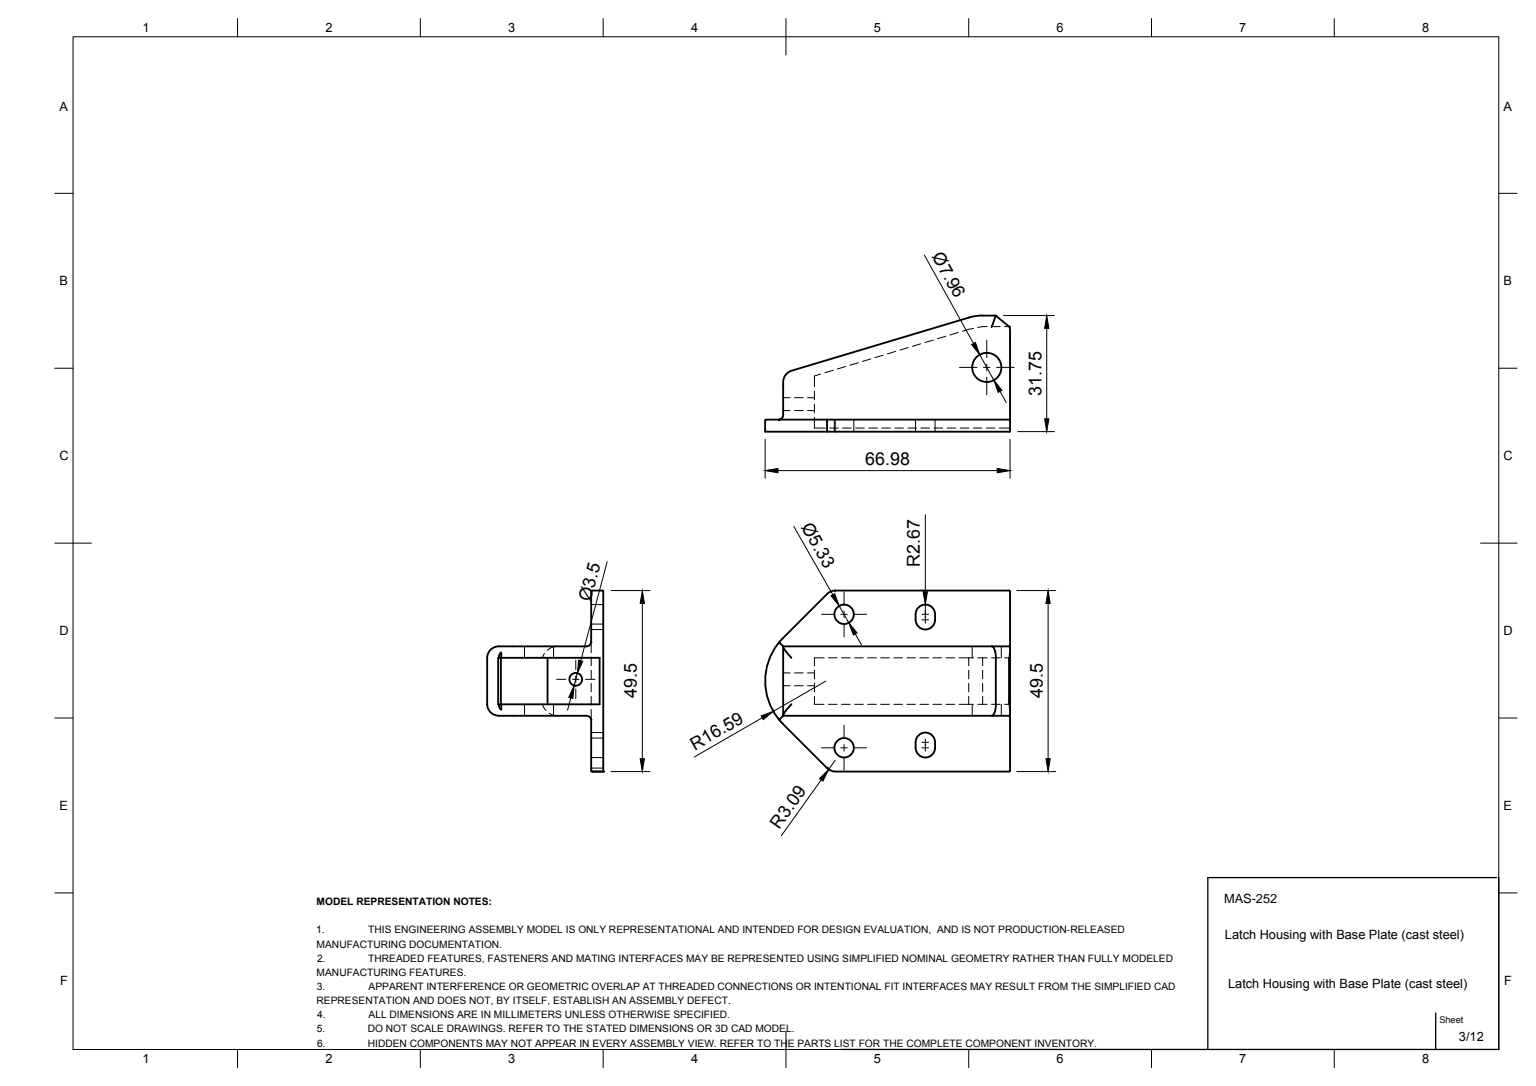
ISO-10303-21;
HEADER;
FILE_DESCRIPTION((''),'2;1');
FILE_NAME('Latch Housing with Base Plate (cast steel).step','2026-10-06T07:01:46+05:00',(''),(''),'','','');
FILE_SCHEMA (('AUTOMOTIVE_DESIGN { 1 0 10303 214 3 1 1 }'));
ENDSEC;
DATA;
#10=MECHANICAL_DESIGN_GEOMETRIC_PRESENTATION_REPRESENTATION('',(#138),#11396);
#108=SHAPE_REPRESENTATION_RELATIONSHIP('SRR','None',#11455,#123) ;
#123=ADVANCED_BREP_SHAPE_REPRESENTATION('',(#153),#11381) ;
#138=STYLED_ITEM('',(#11539),#153) ;
#153=MANIFOLD_SOLID_BREP('Latch Housing with Base Plate (cast steel)',#5569) ;
#168=SPHERICAL_SURFACE('',#5868,0.25) ;
#169=SPHERICAL_SURFACE('',#5870,0.25) ;
#170=B_SPLINE_SURFACE_WITH_KNOTS('',3,3,((#8352,#8353,#8354,#8355,#8356),
(#8357,#8358,#8359,#8360,#8361),(#8362,#8363,#8364,#8365,#8366),(#8367,
#8368,#8369,#8370,#8371),(#8372,#8373,#8374,#8375,#8376)),.UNSPECIFIED.,
 .F.,.F.,.F.,(4,1,4),(4,1,4),(0.,0.5,1.),(0.152021076009298,0.962749790743926,
1.5707963267949),.UNSPECIFIED.) ;
#171=B_SPLINE_SURFACE_WITH_KNOTS('',3,3,((#8498,#8499,#8500,#8501),(#8502,
#8503,#8504,#8505),(#8506,#8507,#8508,#8509),(#8510,#8511,#8512,#8513),
(#8514,#8515,#8516,#8517)),.UNSPECIFIED.,.F.,.F.,.F.,(4,1,4),(4,4),(0.,
0.5,1.),(0.247286151692027,0.297678176745857),.UNSPECIFIED.) ;
#172=B_SPLINE_SURFACE_WITH_KNOTS('',3,3,((#8566,#8567,#8568,#8569),(#8570,
#8571,#8572,#8573),(#8574,#8575,#8576,#8577),(#8578,#8579,#8580,#8581),
(#8582,#8583,#8584,#8585)),.UNSPECIFIED.,.F.,.F.,.F.,(4,1,4),(4,4),(0.,
0.5,1.),(0.268639752323811,0.328790837661693),.UNSPECIFIED.) ;
#173=B_SPLINE_SURFACE_WITH_KNOTS('',3,3,((#8636,#8637,#8638,#8639),(#8640,
#8641,#8642,#8643),(#8644,#8645,#8646,#8647),(#8648,#8649,#8650,#8651),
(#8652,#8653,#8654,#8655)),.UNSPECIFIED.,.F.,.F.,.F.,(4,1,4),(4,4),(0.,
0.5,1.),(8.83098018298437E-16,0.0601510853378708),.UNSPECIFIED.) ;
#174=B_SPLINE_SURFACE_WITH_KNOTS('',3,3,((#8668,#8669,#8670,#8671),(#8672,
#8673,#8674,#8675),(#8676,#8677,#8678,#8679),(#8680,#8681,#8682,#8683),
(#8684,#8685,#8686,#8687)),.UNSPECIFIED.,.F.,.F.,.F.,(4,1,4),(4,4),(0.,
0.5,1.),(1.40103212881273E-16,0.0503920250538296),.UNSPECIFIED.) ;
#175=B_SPLINE_SURFACE_WITH_KNOTS('',3,3,((#8744,#8745,#8746,#8747,#8748),
(#8749,#8750,#8751,#8752,#8753),(#8754,#8755,#8756,#8757,#8758),(#8759,
#8760,#8761,#8762,#8763),(#8764,#8765,#8766,#8767,#8768)),.UNSPECIFIED.,
 .F.,.F.,.F.,(4,1,4),(4,1,4),(0.,0.5,1.),(-1.5707963267949,-0.962749790743935,
-0.152021076009317),.UNSPECIFIED.) ;
#176=TOROIDAL_SURFACE('',#5776,2.915,0.25) ;
#177=TOROIDAL_SURFACE('',#5783,2.915,0.25) ;
#178=TOROIDAL_SURFACE('',#5795,2.915,0.25) ;
#179=TOROIDAL_SURFACE('',#5801,2.915,0.25) ;
#180=TOROIDAL_SURFACE('',#5813,2.915,0.25) ;
#181=TOROIDAL_SURFACE('',#5819,2.915,0.25) ;
#182=TOROIDAL_SURFACE('',#5833,1.52,0.25) ;
#183=TOROIDAL_SURFACE('',#5836,3.05499364382027,0.25) ;
#184=TOROIDAL_SURFACE('',#5838,2.83595375255767,0.25) ;
#185=TOROIDAL_SURFACE('',#5843,16.3358074534161,0.25) ;
#186=TOROIDAL_SURFACE('',#5847,16.3358074534161,0.25) ;
#187=TOROIDAL_SURFACE('',#5850,16.3358074534161,0.25) ;
#188=TOROIDAL_SURFACE('',#5860,1.52,0.25) ;
#189=TOROIDAL_SURFACE('',#5885,10.1848235398934,3.175) ;
#190=TOROIDAL_SURFACE('',#5899,10.1848235398934,3.175) ;
#238=B_SPLINE_CURVE_WITH_KNOTS('',3,(#8214,#8215,#8216,#8217,#8218,#8219,
#8220,#8221,#8222,#8223,#8224,#8225,#8226,#8227,#8228,#8229,#8230,#8231,
#8232,#8233),.UNSPECIFIED.,.F.,.F.,(4,2,2,2,2,2,2,2,2,4),(0.,0.0540586324971382,
0.123044542764543,0.150581892580095,0.158718681491189,0.16330566431825,
0.166396075956513,0.169257252570085,0.172939173780484,0.178310039493042),
 .UNSPECIFIED.) ;
#239=B_SPLINE_CURVE_WITH_KNOTS('',3,(#8399,#8400,#8401,#8402,#8403,#8404,
#8405,#8406,#8407,#8408,#8409,#8410,#8411,#8412,#8413,#8414,#8415,#8416,
#8417,#8418,#8419,#8420,#8421,#8422,#8423,#8424,#8425,#8426),
 .UNSPECIFIED.,.F.,.F.,(4,3,3,3,3,3,3,3,3,4),(0.,0.196349544517553,0.384559246386717,
0.572733492677506,0.76087751170374,0.948996522878222,1.13718101963994,1.32530709535773,
1.51344876765349,1.57079635614042),.UNSPECIFIED.) ;
#240=B_SPLINE_CURVE_WITH_KNOTS('',3,(#8427,#8428,#8429,#8430,#8431,#8432,
#8433,#8434,#8435,#8436,#8437,#8438),.UNSPECIFIED.,.F.,.F.,(4,2,2,2,2,4),
(-0.000461918039195691,0.,0.00963254585094742,0.0193990205733435,0.0291649301246413,
0.0389305592704718),.UNSPECIFIED.) ;
#241=B_SPLINE_CURVE_WITH_KNOTS('',3,(#8441,#8442,#8443,#8444,#8445,#8446,
#8447,#8448,#8449,#8450,#8451,#8452,#8453,#8454,#8455,#8456,#8457,#8458,
#8459,#8460,#8461,#8462,#8463,#8464,#8465,#8466,#8467,#8468),
 .UNSPECIFIED.,.F.,.F.,(4,3,3,3,3,3,3,3,3,4),(0.,0.196349545007139,0.384559245883083,
0.57273349111916,0.760877509017182,0.94899651898573,1.13718101444157,1.32530708880429,
1.51344875970823,1.57079636005712),.UNSPECIFIED.) ;
#242=B_SPLINE_CURVE_WITH_KNOTS('',3,(#8470,#8471,#8472,#8473,#8474,#8475,
#8476,#8477,#8478,#8479,#8480,#8481),.UNSPECIFIED.,.F.,.F.,(4,2,2,2,2,4),
(-0.0393922331407002,-0.0389148464755049,-0.0292979433455524,-0.019531495885866,
-0.00976560909452869,0.),.UNSPECIFIED.) ;
#243=B_SPLINE_CURVE_WITH_KNOTS('',3,(#8485,#8486,#8487,#8488,#8489,#8490,
#8491,#8492,#8493,#8494,#8495,#8496),.UNSPECIFIED.,.F.,.F.,(4,2,2,2,2,4),
(-0.0393901610897999,-0.0388026611771767,-0.0292983305555518,-0.0195322143643491,
-0.00976610536427336,0.),.UNSPECIFIED.) ;
#244=B_SPLINE_CURVE_WITH_KNOTS('',3,(#8519,#8520,#8521,#8522),
 .UNSPECIFIED.,.F.,.F.,(4,4),(0.247286151692027,0.297678176745857),
 .UNSPECIFIED.) ;
#245=B_SPLINE_CURVE_WITH_KNOTS('',3,(#8526,#8527,#8528,#8529),
 .UNSPECIFIED.,.F.,.F.,(4,4),(-0.297678176745857,-0.251823353043443),
 .UNSPECIFIED.) ;
#246=B_SPLINE_CURVE_WITH_KNOTS('',3,(#8531,#8532,#8533,#8534,#8535,#8536,
#8537,#8538,#8539,#8540,#8541,#8542,#8543,#8544,#8545,#8546,#8547,#8548,
#8549,#8550,#8551,#8552,#8553,#8554,#8555,#8556,#8557,#8558,#8559,#8560,
#8561),.UNSPECIFIED.,.F.,.F.,(4,3,3,3,3,3,3,3,3,3,4),(-0.0348625063534064,
-0.0346987118982289,-0.0299534938780202,-0.0270418791157803,-0.0222988095360682,
-0.0194379956728184,-0.0169333679581277,-0.0122101103613041,-0.00963834412463436,
-0.00481917206231718,0.),.UNSPECIFIED.) ;
#247=B_SPLINE_CURVE_WITH_KNOTS('',3,(#8562,#8563,#8564,#8565),
 .UNSPECIFIED.,.F.,.F.,(4,4),(0.0910103417204836,0.0923523226751523),
 .UNSPECIFIED.) ;
#248=B_SPLINE_CURVE_WITH_KNOTS('',3,(#8588,#8589,#8590,#8591),
 .UNSPECIFIED.,.F.,.F.,(4,4),(0.268639752323811,0.328790837661693),
 .UNSPECIFIED.) ;
#249=B_SPLINE_CURVE_WITH_KNOTS('',3,(#8595,#8596,#8597,#8598),
 .UNSPECIFIED.,.F.,.F.,(4,4),(-0.328790837661693,-0.273035259145455),
 .UNSPECIFIED.) ;
#250=B_SPLINE_CURVE_WITH_KNOTS('',3,(#8599,#8600,#8601,#8602,#8603,#8604,
#8605,#8606,#8607,#8608,#8609,#8610,#8611,#8612,#8613,#8614,#8615,#8616,
#8617,#8618,#8619,#8620,#8621,#8622,#8623,#8624,#8625,#8626,#8627,#8628,
#8629),.UNSPECIFIED.,.F.,.F.,(4,3,3,3,3,3,3,3,3,3,4),(-0.000163872705022366,
0.,0.00475051443863407,0.00766049069720532,0.0124072603708054,0.0152680067602041,
0.017390180489341,0.0221174050715347,0.0250723399175726,0.0298938142536046,
0.0347152885896365),.UNSPECIFIED.) ;
#251=B_SPLINE_CURVE_WITH_KNOTS('',3,(#8656,#8657,#8658,#8659),
 .UNSPECIFIED.,.F.,.F.,(4,4),(-0.0557555785162243,-8.83098018298437E-16),
 .UNSPECIFIED.) ;
#252=B_SPLINE_CURVE_WITH_KNOTS('',3,(#8660,#8661,#8662,#8663),
 .UNSPECIFIED.,.F.,.F.,(4,4),(8.83098018298437E-16,0.0601510853378708),
 .UNSPECIFIED.) ;
#253=B_SPLINE_CURVE_WITH_KNOTS('',3,(#8688,#8689,#8690,#8691),
 .UNSPECIFIED.,.F.,.F.,(4,4),(-0.0458548237024101,-1.40103212881273E-16),
 .UNSPECIFIED.) ;
#254=B_SPLINE_CURVE_WITH_KNOTS('',3,(#8693,#8694,#8695,#8696),
 .UNSPECIFIED.,.F.,.F.,(4,4),(1.40103212881273E-16,0.0503920250538296),
 .UNSPECIFIED.) ;
#255=B_SPLINE_CURVE_WITH_KNOTS('',3,(#8697,#8698,#8699,#8700),
 .UNSPECIFIED.,.F.,.F.,(4,4),(0.,0.00076501868574839),.UNSPECIFIED.) ;
#256=B_SPLINE_CURVE_WITH_KNOTS('',3,(#8704,#8705,#8706,#8707,#8708,#8709,
#8710,#8711,#8712,#8713,#8714,#8715),.UNSPECIFIED.,.F.,.F.,(4,2,2,2,2,4),
(-0.00058749989859564,0.,0.00950433039685776,0.019270446358007,0.0290365551280728,
0.0388026602624192),.UNSPECIFIED.) ;
#257=B_SPLINE_CURVE_WITH_KNOTS('',3,(#8771,#8772,#8773,#8774,#8775,#8776,
#8777,#8778,#8779,#8780,#8781,#8782,#8783,#8784,#8785,#8786,#8787,#8788,
#8789,#8790),.UNSPECIFIED.,.F.,.F.,(4,2,2,2,2,2,2,2,2,4),(0.,0.00187316890925574,
0.00298322418909923,0.00385163372182826,0.00475787590428727,0.00612708715977988,
0.00905111735916402,0.0164269109230864,0.0329222866646951,0.0555625738155659),
 .UNSPECIFIED.) ;
#258=B_SPLINE_CURVE_WITH_KNOTS('',3,(#8834,#8835,#8836,#8837,#8838,#8839,
#8840,#8841,#8842,#8843,#8844,#8845,#8846,#8847,#8848,#8849,#8850,#8851,
#8852,#8853,#8854,#8855,#8856,#8857,#8858,#8859,#8860,#8861,#8862,#8863,
#8864,#8865,#8866,#8867,#8868,#8869,#8870,#8871,#8872,#8873,#8874,#8875,
#8876,#8877,#8878,#8879,#8880,#8881,#8882),.UNSPECIFIED.,.F.,.F.,(4,3,3,
3,3,3,3,3,3,3,3,3,3,3,3,3,4),(0.,0.09964938522947,0.199295818282578,0.298939491768606,
0.39858059832873,0.498219330669901,0.597855881594742,0.697490444026332,
0.797123211027307,0.896771849198539,0.996414865845315,1.09605303531753,
1.19568713170185,1.29533435965265,1.39497149040076,1.4946160591622,1.57079725751296),
 .UNSPECIFIED.) ;
#259=B_SPLINE_CURVE_WITH_KNOTS('',3,(#8883,#8884,#8885,#8886,#8887,#8888,
#8889,#8890,#8891,#8892,#8893,#8894,#8895,#8896,#8897,#8898,#8899,#8900),
 .UNSPECIFIED.,.F.,.F.,(4,2,2,2,2,2,2,2,4),(-0.00724818355843104,0.,0.00866972814024576,
0.0246774186784591,0.0566526412437171,0.120620928432891,0.244650657098656,
0.368680208659511,0.492709676950837),.UNSPECIFIED.) ;
#260=B_SPLINE_CURVE_WITH_KNOTS('',3,(#8907,#8908,#8909,#8910,#8911,#8912,
#8913,#8914,#8915,#8916,#8917,#8918,#8919,#8920,#8921,#8922,#8923,#8924,
#8925,#8926,#8927,#8928),.UNSPECIFIED.,.F.,.F.,(4,2,2,2,2,2,2,2,2,2,4),
(0.656794478552693,0.697723395150039,0.83000632281984,1.01882918615295,
1.1132406178195,1.16044633365278,1.18404919156942,1.19585062052774,1.2017513350069,
1.20470169224648,1.20765204948606),.UNSPECIFIED.) ;
#261=B_SPLINE_CURVE_WITH_KNOTS('',3,(#8947,#8948,#8949,#8950,#8951,#8952,
#8953,#8954,#8955,#8956,#8957,#8958,#8959,#8960,#8961,#8962,#8963,#8964,
#8965,#8966,#8967,#8968),.UNSPECIFIED.,.F.,.F.,(4,2,2,2,2,2,2,2,2,2,4),
(1.20765204948607,1.21060240672565,1.21355276396523,1.21945347844439,1.2312549074027,
1.25485776531934,1.30206348115262,1.39647491281918,1.58529777615229,1.71758070382209,
1.75850962041944),.UNSPECIFIED.) ;
#262=B_SPLINE_CURVE_WITH_KNOTS('',3,(#8971,#8972,#8973,#8974,#8975,#8976,
#8977,#8978,#8979,#8980,#8981,#8982,#8983,#8984,#8985,#8986,#8987,#8988),
 .UNSPECIFIED.,.F.,.F.,(4,2,2,2,2,2,2,2,4),(-0.499957830797754,-0.492709647672271,
-0.484039920050198,-0.468032230464552,-0.436057009799713,-0.372088726411136,
-0.248059005111197,-0.124029460922085,0.),.UNSPECIFIED.) ;
#263=B_SPLINE_CURVE_WITH_KNOTS('',3,(#8990,#8991,#8992,#8993,#8994,#8995,
#8996,#8997,#8998,#8999,#9000,#9001,#9002,#9003,#9004,#9005,#9006,#9007,
#9008,#9009,#9010,#9011,#9012,#9013,#9014,#9015,#9016,#9017,#9018,#9019,
#9020,#9021,#9022,#9023,#9024,#9025,#9026,#9027,#9028,#9029,#9030,#9031,
#9032,#9033,#9034,#9035,#9036,#9037,#9038),.UNSPECIFIED.,.F.,.F.,(4,3,3,
3,3,3,3,3,3,3,3,3,3,3,3,3,4),(0.,0.0996501112039543,0.199297271810784,0.298941675382784,
0.398583515425884,0.498222985393558,0.597860278690689,0.697495588677662,
0.797129108674119,0.896778508053707,0.996422290829433,1.09606123100929,
1.19569610220027,1.29534410980026,1.39498202233642,1.4946273745031,1.57080590414797),
 .UNSPECIFIED.) ;
#337=FACE_BOUND('',#849,.T.) ;
#338=FACE_BOUND('',#853,.T.) ;
#339=FACE_BOUND('',#856,.T.) ;
#340=FACE_BOUND('',#867,.T.) ;
#341=FACE_BOUND('',#868,.T.) ;
#342=FACE_BOUND('',#873,.T.) ;
#343=FACE_BOUND('',#874,.T.) ;
#344=FACE_BOUND('',#906,.T.) ;
#345=FACE_BOUND('',#912,.T.) ;
#346=FACE_BOUND('',#926,.T.) ;
#347=FACE_BOUND('',#942,.T.) ;
#348=FACE_BOUND('',#943,.T.) ;
#349=FACE_BOUND('',#944,.T.) ;
#350=FACE_BOUND('',#945,.T.) ;
#378=ELLIPSE('',#5762,4.97501164804779,3.175) ;
#379=ELLIPSE('',#5763,4.97501164804779,3.175) ;
#380=ELLIPSE('',#5772,4.72548959035073,3.175) ;
#381=ELLIPSE('',#5773,3.9949536559852,3.175) ;
#382=ELLIPSE('',#5774,3.37510195454879,3.175) ;
#383=ELLIPSE('',#5826,3.79929660772484,2.925) ;
#384=ELLIPSE('',#5866,3.9949536559852,3.175) ;
#385=ELLIPSE('',#5867,3.79929660772485,2.925) ;
#386=ELLIPSE('',#5875,1.79605122421383,1.27) ;
#387=ELLIPSE('',#5878,1.79605122421383,1.27) ;
#388=ELLIPSE('',#5883,3.37510195454879,3.175) ;
#389=ELLIPSE('',#5884,4.72548959035073,3.175) ;
#390=ELLIPSE('',#5889,3.3147973165791,3.175) ;
#391=ELLIPSE('',#5897,3.3147973165791,3.175) ;
#396=PLANE('',#5761) ;
#397=PLANE('',#5764) ;
#398=PLANE('',#5765) ;
#399=PLANE('',#5766) ;
#400=PLANE('',#5767) ;
#401=PLANE('',#5768) ;
#402=PLANE('',#5769) ;
#403=PLANE('',#5770) ;
#404=PLANE('',#5775) ;
#405=PLANE('',#5788) ;
#406=PLANE('',#5791) ;
#407=PLANE('',#5806) ;
#408=PLANE('',#5823) ;
#409=PLANE('',#5872) ;
#410=PLANE('',#5876) ;
#411=PLANE('',#5880) ;
#412=PLANE('',#5890) ;
#413=PLANE('',#5891) ;
#414=PLANE('',#5894) ;
#415=PLANE('',#5900) ;
#416=PLANE('',#5901) ;
#417=PLANE('',#5904) ;
#418=PLANE('',#5907) ;
#419=PLANE('',#5910) ;
#420=PLANE('',#5913) ;
#421=PLANE('',#5916) ;
#422=PLANE('',#5919) ;
#423=PLANE('',#5922) ;
#508=FACE_OUTER_BOUND('',#844,.T.) ;
#509=FACE_OUTER_BOUND('',#845,.T.) ;
#510=FACE_OUTER_BOUND('',#846,.T.) ;
#511=FACE_OUTER_BOUND('',#847,.T.) ;
#512=FACE_OUTER_BOUND('',#848,.T.) ;
#513=FACE_OUTER_BOUND('',#850,.T.) ;
#514=FACE_OUTER_BOUND('',#851,.T.) ;
#515=FACE_OUTER_BOUND('',#852,.T.) ;
#516=FACE_OUTER_BOUND('',#854,.T.) ;
#517=FACE_OUTER_BOUND('',#855,.T.) ;
#518=FACE_OUTER_BOUND('',#857,.T.) ;
#519=FACE_OUTER_BOUND('',#858,.T.) ;
#520=FACE_OUTER_BOUND('',#859,.T.) ;
#521=FACE_OUTER_BOUND('',#860,.T.) ;
#522=FACE_OUTER_BOUND('',#861,.T.) ;
#523=FACE_OUTER_BOUND('',#862,.T.) ;
#524=FACE_OUTER_BOUND('',#863,.T.) ;
#525=FACE_OUTER_BOUND('',#864,.T.) ;
#526=FACE_OUTER_BOUND('',#865,.T.) ;
#527=FACE_OUTER_BOUND('',#866,.T.) ;
#528=FACE_OUTER_BOUND('',#869,.T.) ;
#529=FACE_OUTER_BOUND('',#870,.T.) ;
#530=FACE_OUTER_BOUND('',#871,.T.) ;
#531=FACE_OUTER_BOUND('',#872,.T.) ;
#532=FACE_OUTER_BOUND('',#875,.T.) ;
#533=FACE_OUTER_BOUND('',#876,.T.) ;
#534=FACE_OUTER_BOUND('',#877,.T.) ;
#535=FACE_OUTER_BOUND('',#878,.T.) ;
#536=FACE_OUTER_BOUND('',#879,.T.) ;
#537=FACE_OUTER_BOUND('',#880,.T.) ;
#538=FACE_OUTER_BOUND('',#881,.T.) ;
#539=FACE_OUTER_BOUND('',#882,.T.) ;
#540=FACE_OUTER_BOUND('',#883,.T.) ;
#541=FACE_OUTER_BOUND('',#884,.T.) ;
#542=FACE_OUTER_BOUND('',#885,.T.) ;
#543=FACE_OUTER_BOUND('',#886,.T.) ;
#544=FACE_OUTER_BOUND('',#887,.T.) ;
#545=FACE_OUTER_BOUND('',#888,.T.) ;
#546=FACE_OUTER_BOUND('',#889,.T.) ;
#547=FACE_OUTER_BOUND('',#890,.T.) ;
#548=FACE_OUTER_BOUND('',#891,.T.) ;
#549=FACE_OUTER_BOUND('',#892,.T.) ;
#550=FACE_OUTER_BOUND('',#893,.T.) ;
#551=FACE_OUTER_BOUND('',#894,.T.) ;
#552=FACE_OUTER_BOUND('',#895,.T.) ;
#553=FACE_OUTER_BOUND('',#896,.T.) ;
#554=FACE_OUTER_BOUND('',#897,.T.) ;
#555=FACE_OUTER_BOUND('',#898,.T.) ;
#556=FACE_OUTER_BOUND('',#899,.T.) ;
#557=FACE_OUTER_BOUND('',#900,.T.) ;
#558=FACE_OUTER_BOUND('',#901,.T.) ;
#559=FACE_OUTER_BOUND('',#902,.T.) ;
#560=FACE_OUTER_BOUND('',#903,.T.) ;
#561=FACE_OUTER_BOUND('',#904,.T.) ;
#562=FACE_OUTER_BOUND('',#905,.T.) ;
#563=FACE_OUTER_BOUND('',#907,.T.) ;
#564=FACE_OUTER_BOUND('',#908,.T.) ;
#565=FACE_OUTER_BOUND('',#909,.T.) ;
#566=FACE_OUTER_BOUND('',#910,.T.) ;
#567=FACE_OUTER_BOUND('',#911,.T.) ;
#568=FACE_OUTER_BOUND('',#913,.T.) ;
#569=FACE_OUTER_BOUND('',#914,.T.) ;
#570=FACE_OUTER_BOUND('',#915,.T.) ;
#571=FACE_OUTER_BOUND('',#916,.T.) ;
#572=FACE_OUTER_BOUND('',#917,.T.) ;
#573=FACE_OUTER_BOUND('',#918,.T.) ;
#574=FACE_OUTER_BOUND('',#919,.T.) ;
#575=FACE_OUTER_BOUND('',#920,.T.) ;
#576=FACE_OUTER_BOUND('',#921,.T.) ;
#577=FACE_OUTER_BOUND('',#922,.T.) ;
#578=FACE_OUTER_BOUND('',#923,.T.) ;
#579=FACE_OUTER_BOUND('',#924,.T.) ;
#580=FACE_OUTER_BOUND('',#925,.T.) ;
#581=FACE_OUTER_BOUND('',#927,.T.) ;
#582=FACE_OUTER_BOUND('',#928,.T.) ;
#583=FACE_OUTER_BOUND('',#929,.T.) ;
#584=FACE_OUTER_BOUND('',#930,.T.) ;
#585=FACE_OUTER_BOUND('',#931,.T.) ;
#586=FACE_OUTER_BOUND('',#932,.T.) ;
#587=FACE_OUTER_BOUND('',#933,.T.) ;
#588=FACE_OUTER_BOUND('',#934,.T.) ;
#589=FACE_OUTER_BOUND('',#935,.T.) ;
#590=FACE_OUTER_BOUND('',#936,.T.) ;
#591=FACE_OUTER_BOUND('',#937,.T.) ;
#592=FACE_OUTER_BOUND('',#938,.T.) ;
#593=FACE_OUTER_BOUND('',#939,.T.) ;
#594=FACE_OUTER_BOUND('',#940,.T.) ;
#595=FACE_OUTER_BOUND('',#941,.T.) ;
#844=EDGE_LOOP('',(#3528,#3529,#3530,#3531)) ;
#845=EDGE_LOOP('',(#3532,#3533,#3534,#3535)) ;
#846=EDGE_LOOP('',(#3536,#3537,#3538,#3539)) ;
#847=EDGE_LOOP('',(#3540,#3541,#3542,#3543,#3544,#3545)) ;
#848=EDGE_LOOP('',(#3546,#3547,#3548,#3549,#3550,#3551,#3552,#3553)) ;
#849=EDGE_LOOP('',(#3554)) ;
#850=EDGE_LOOP('',(#3555,#3556,#3557,#3558)) ;
#851=EDGE_LOOP('',(#3559,#3560,#3561,#3562)) ;
#852=EDGE_LOOP('',(#3563,#3564,#3565,#3566)) ;
#853=EDGE_LOOP('',(#3567)) ;
#854=EDGE_LOOP('',(#3568,#3569,#3570,#3571)) ;
#855=EDGE_LOOP('',(#3572,#3573,#3574,#3575,#3576,#3577,#3578,#3579)) ;
#856=EDGE_LOOP('',(#3580)) ;
#857=EDGE_LOOP('',(#3581,#3582,#3583,#3584)) ;
#858=EDGE_LOOP('',(#3585,#3586,#3587,#3588,#3589,#3590,#3591)) ;
#859=EDGE_LOOP('',(#3592,#3593,#3594,#3595)) ;
#860=EDGE_LOOP('',(#3596,#3597,#3598,#3599)) ;
#861=EDGE_LOOP('',(#3600,#3601,#3602,#3603)) ;
#862=EDGE_LOOP('',(#3604,#3605,#3606,#3607)) ;
#863=EDGE_LOOP('',(#3608,#3609,#3610,#3611)) ;
#864=EDGE_LOOP('',(#3612,#3613,#3614,#3615)) ;
#865=EDGE_LOOP('',(#3616,#3617,#3618,#3619)) ;
#866=EDGE_LOOP('',(#3620,#3621,#3622,#3623,#3624,#3625)) ;
#867=EDGE_LOOP('',(#3626)) ;
#868=EDGE_LOOP('',(#3627,#3628,#3629,#3630)) ;
#869=EDGE_LOOP('',(#3631,#3632,#3633,#3634,#3635)) ;
#870=EDGE_LOOP('',(#3636,#3637,#3638,#3639,#3640)) ;
#871=EDGE_LOOP('',(#3641,#3642,#3643,#3644,#3645)) ;
#872=EDGE_LOOP('',(#3646,#3647,#3648,#3649,#3650,#3651)) ;
#873=EDGE_LOOP('',(#3652,#3653,#3654,#3655)) ;
#874=EDGE_LOOP('',(#3656)) ;
#875=EDGE_LOOP('',(#3657,#3658,#3659,#3660,#3661)) ;
#876=EDGE_LOOP('',(#3662,#3663,#3664,#3665)) ;
#877=EDGE_LOOP('',(#3666,#3667,#3668,#3669)) ;
#878=EDGE_LOOP('',(#3670,#3671,#3672,#3673)) ;
#879=EDGE_LOOP('',(#3674,#3675,#3676,#3677)) ;
#880=EDGE_LOOP('',(#3678,#3679,#3680,#3681)) ;
#881=EDGE_LOOP('',(#3682,#3683,#3684,#3685)) ;
#882=EDGE_LOOP('',(#3686,#3687,#3688,#3689)) ;
#883=EDGE_LOOP('',(#3690,#3691,#3692,#3693)) ;
#884=EDGE_LOOP('',(#3694,#3695,#3696,#3697)) ;
#885=EDGE_LOOP('',(#3698,#3699,#3700,#3701)) ;
#886=EDGE_LOOP('',(#3702,#3703,#3704,#3705)) ;
#887=EDGE_LOOP('',(#3706,#3707,#3708,#3709)) ;
#888=EDGE_LOOP('',(#3710,#3711,#3712,#3713)) ;
#889=EDGE_LOOP('',(#3714,#3715,#3716,#3717,#3718)) ;
#890=EDGE_LOOP('',(#3719,#3720,#3721,#3722)) ;
#891=EDGE_LOOP('',(#3723,#3724,#3725,#3726)) ;
#892=EDGE_LOOP('',(#3727,#3728,#3729,#3730)) ;
#893=EDGE_LOOP('',(#3731,#3732,#3733,#3734)) ;
#894=EDGE_LOOP('',(#3735,#3736,#3737,#3738,#3739)) ;
#895=EDGE_LOOP('',(#3740,#3741,#3742,#3743)) ;
#896=EDGE_LOOP('',(#3744,#3745,#3746,#3747)) ;
#897=EDGE_LOOP('',(#3748,#3749,#3750,#3751)) ;
#898=EDGE_LOOP('',(#3752,#3753,#3754,#3755)) ;
#899=EDGE_LOOP('',(#3756,#3757,#3758,#3759)) ;
#900=EDGE_LOOP('',(#3760,#3761,#3762,#3763)) ;
#901=EDGE_LOOP('',(#3764,#3765,#3766,#3767)) ;
#902=EDGE_LOOP('',(#3768,#3769,#3770,#3771)) ;
#903=EDGE_LOOP('',(#3772,#3773,#3774)) ;
#904=EDGE_LOOP('',(#3775,#3776,#3777)) ;
#905=EDGE_LOOP('',(#3778,#3779,#3780,#3781,#3782,#3783,#3784)) ;
#906=EDGE_LOOP('',(#3785)) ;
#907=EDGE_LOOP('',(#3786,#3787,#3788,#3789,#3790)) ;
#908=EDGE_LOOP('',(#3791,#3792)) ;
#909=EDGE_LOOP('',(#3793,#3794,#3795,#3796,#3797,#3798,#3799,#3800)) ;
#910=EDGE_LOOP('',(#3801,#3802,#3803,#3804,#3805)) ;
#911=EDGE_LOOP('',(#3806,#3807,#3808,#3809,#3810,#3811,#3812)) ;
#912=EDGE_LOOP('',(#3813)) ;
#913=EDGE_LOOP('',(#3814,#3815,#3816,#3817,#3818,#3819,#3820)) ;
#914=EDGE_LOOP('',(#3821,#3822,#3823,#3824)) ;
#915=EDGE_LOOP('',(#3825,#3826,#3827,#3828)) ;
#916=EDGE_LOOP('',(#3829,#3830,#3831,#3832,#3833)) ;
#917=EDGE_LOOP('',(#3834,#3835,#3836,#3837)) ;
#918=EDGE_LOOP('',(#3838,#3839,#3840,#3841)) ;
#919=EDGE_LOOP('',(#3842,#3843,#3844,#3845)) ;
#920=EDGE_LOOP('',(#3846,#3847,#3848,#3849)) ;
#921=EDGE_LOOP('',(#3850,#3851,#3852,#3853)) ;
#922=EDGE_LOOP('',(#3854,#3855,#3856,#3857,#3858)) ;
#923=EDGE_LOOP('',(#3859,#3860,#3861,#3862)) ;
#924=EDGE_LOOP('',(#3863,#3864,#3865,#3866)) ;
#925=EDGE_LOOP('',(#3867,#3868,#3869,#3870,#3871,#3872)) ;
#926=EDGE_LOOP('',(#3873)) ;
#927=EDGE_LOOP('',(#3874,#3875,#3876,#3877)) ;
#928=EDGE_LOOP('',(#3878,#3879,#3880,#3881)) ;
#929=EDGE_LOOP('',(#3882,#3883,#3884,#3885)) ;
#930=EDGE_LOOP('',(#3886,#3887,#3888,#3889)) ;
#931=EDGE_LOOP('',(#3890,#3891,#3892,#3893)) ;
#932=EDGE_LOOP('',(#3894,#3895,#3896,#3897)) ;
#933=EDGE_LOOP('',(#3898,#3899,#3900,#3901)) ;
#934=EDGE_LOOP('',(#3902,#3903,#3904,#3905,#3906,#3907,#3908,#3909,#3910,
#3911)) ;
#935=EDGE_LOOP('',(#3912,#3913,#3914,#3915)) ;
#936=EDGE_LOOP('',(#3916,#3917,#3918,#3919)) ;
#937=EDGE_LOOP('',(#3920,#3921,#3922,#3923)) ;
#938=EDGE_LOOP('',(#3924,#3925,#3926,#3927)) ;
#939=EDGE_LOOP('',(#3928,#3929,#3930,#3931,#3932,#3933,#3934,#3935,#3936,
#3937,#3938,#3939,#3940,#3941,#3942,#3943)) ;
#940=EDGE_LOOP('',(#3944,#3945,#3946,#3947)) ;
#941=EDGE_LOOP('',(#3948,#3949,#3950,#3951,#3952,#3953,#3954,#3955,#3956,
#3957)) ;
#942=EDGE_LOOP('',(#3958)) ;
#943=EDGE_LOOP('',(#3959,#3960,#3961,#3962)) ;
#944=EDGE_LOOP('',(#3963)) ;
#945=EDGE_LOOP('',(#3964,#3965,#3966,#3967)) ;
#1221=LINE('',#8134,#1604) ;
#1222=LINE('',#8140,#1605) ;
#1223=LINE('',#8146,#1606) ;
#1224=LINE('',#8153,#1607) ;
#1225=LINE('',#8155,#1608) ;
#1226=LINE('',#8157,#1609) ;
#1227=LINE('',#8160,#1610) ;
#1228=LINE('',#8163,#1611) ;
#1229=LINE('',#8165,#1612) ;
#1230=LINE('',#8167,#1613) ;
#1231=LINE('',#8169,#1614) ;
#1232=LINE('',#8171,#1615) ;
#1233=LINE('',#8173,#1616) ;
#1234=LINE('',#8174,#1617) ;
#1235=LINE('',#8177,#1618) ;
#1236=LINE('',#8178,#1619) ;
#1237=LINE('',#8181,#1620) ;
#1238=LINE('',#8182,#1621) ;
#1239=LINE('',#8185,#1622) ;
#1240=LINE('',#8186,#1623) ;
#1241=LINE('',#8189,#1624) ;
#1242=LINE('',#8190,#1625) ;
#1243=LINE('',#8193,#1626) ;
#1244=LINE('',#8195,#1627) ;
#1245=LINE('',#8196,#1628) ;
#1246=LINE('',#8199,#1629) ;
#1247=LINE('',#8201,#1630) ;
#1248=LINE('',#8202,#1631) ;
#1249=LINE('',#8209,#1632) ;
#1250=LINE('',#8213,#1633) ;
#1251=LINE('',#8247,#1634) ;
#1252=LINE('',#8248,#1635) ;
#1253=LINE('',#8256,#1636) ;
#1254=LINE('',#8257,#1637) ;
#1255=LINE('',#8260,#1638) ;
#1256=LINE('',#8262,#1639) ;
#1257=LINE('',#8263,#1640) ;
#1258=LINE('',#8266,#1641) ;
#1259=LINE('',#8273,#1642) ;
#1260=LINE('',#8277,#1643) ;
#1261=LINE('',#8279,#1644) ;
#1262=LINE('',#8280,#1645) ;
#1263=LINE('',#8291,#1646) ;
#1264=LINE('',#8304,#1647) ;
#1265=LINE('',#8306,#1648) ;
#1266=LINE('',#8310,#1649) ;
#1267=LINE('',#8313,#1650) ;
#1268=LINE('',#8318,#1651) ;
#1269=LINE('',#8321,#1652) ;
#1270=LINE('',#8324,#1653) ;
#1271=LINE('',#8335,#1654) ;
#1272=LINE('',#8341,#1655) ;
#1273=LINE('',#8344,#1656) ;
#1274=LINE('',#8346,#1657) ;
#1275=LINE('',#8347,#1658) ;
#1276=LINE('',#8350,#1659) ;
#1277=LINE('',#8384,#1660) ;
#1278=LINE('',#8385,#1661) ;
#1279=LINE('',#8390,#1662) ;
#1280=LINE('',#8497,#1663) ;
#1281=LINE('',#8717,#1664) ;
#1282=LINE('',#8720,#1665) ;
#1283=LINE('',#8725,#1666) ;
#1284=LINE('',#8730,#1667) ;
#1285=LINE('',#8742,#1668) ;
#1286=LINE('',#8743,#1669) ;
#1287=LINE('',#8799,#1670) ;
#1288=LINE('',#8801,#1671) ;
#1289=LINE('',#8803,#1672) ;
#1290=LINE('',#8806,#1673) ;
#1291=LINE('',#8810,#1674) ;
#1292=LINE('',#8814,#1675) ;
#1293=LINE('',#8816,#1676) ;
#1294=LINE('',#8819,#1677) ;
#1295=LINE('',#8821,#1678) ;
#1296=LINE('',#8825,#1679) ;
#1297=LINE('',#8826,#1680) ;
#1298=LINE('',#8902,#1681) ;
#1299=LINE('',#8929,#1682) ;
#1300=LINE('',#8931,#1683) ;
#1301=LINE('',#8934,#1684) ;
#1302=LINE('',#8935,#1685) ;
#1303=LINE('',#8938,#1686) ;
#1304=LINE('',#8942,#1687) ;
#1305=LINE('',#8943,#1688) ;
#1306=LINE('',#8946,#1689) ;
#1307=LINE('',#9043,#1690) ;
#1308=LINE('',#9044,#1691) ;
#1309=LINE('',#9049,#1692) ;
#1310=LINE('',#9050,#1693) ;
#1311=LINE('',#9055,#1694) ;
#1312=LINE('',#9057,#1695) ;
#1313=LINE('',#9058,#1696) ;
#1314=LINE('',#9061,#1697) ;
#1315=LINE('',#9065,#1698) ;
#1316=LINE('',#9066,#1699) ;
#1317=LINE('',#9069,#1700) ;
#1318=LINE('',#9073,#1701) ;
#1319=LINE('',#9074,#1702) ;
#1320=LINE('',#9077,#1703) ;
#1321=LINE('',#9081,#1704) ;
#1322=LINE('',#9082,#1705) ;
#1323=LINE('',#9085,#1706) ;
#1324=LINE('',#9089,#1707) ;
#1325=LINE('',#9090,#1708) ;
#1604=VECTOR('',#6423,1.75) ;
#1605=VECTOR('',#6430,3.98) ;
#1606=VECTOR('',#6437,3.98) ;
#1607=VECTOR('',#6444,10.) ;
#1608=VECTOR('',#6445,10.) ;
#1609=VECTOR('',#6446,10.) ;
#1610=VECTOR('',#6449,10.) ;
#1611=VECTOR('',#6452,10.) ;
#1612=VECTOR('',#6453,10.) ;
#1613=VECTOR('',#6454,10.) ;
#1614=VECTOR('',#6455,10.) ;
#1615=VECTOR('',#6456,10.) ;
#1616=VECTOR('',#6457,10.) ;
#1617=VECTOR('',#6458,10.) ;
#1618=VECTOR('',#6461,10.) ;
#1619=VECTOR('',#6462,10.) ;
#1620=VECTOR('',#6465,10.) ;
#1621=VECTOR('',#6466,10.) ;
#1622=VECTOR('',#6469,10.) ;
#1623=VECTOR('',#6470,10.) ;
#1624=VECTOR('',#6473,10.) ;
#1625=VECTOR('',#6474,10.) ;
#1626=VECTOR('',#6477,10.) ;
#1627=VECTOR('',#6478,10.) ;
#1628=VECTOR('',#6479,10.) ;
#1629=VECTOR('',#6482,10.) ;
#1630=VECTOR('',#6483,10.) ;
#1631=VECTOR('',#6484,10.) ;
#1632=VECTOR('',#6491,10.) ;
#1633=VECTOR('',#6496,10.) ;
#1634=VECTOR('',#6511,10.) ;
#1635=VECTOR('',#6512,10.) ;
#1636=VECTOR('',#6523,10.) ;
#1637=VECTOR('',#6524,10.) ;
#1638=VECTOR('',#6527,10.) ;
#1639=VECTOR('',#6528,10.) ;
#1640=VECTOR('',#6529,10.) ;
#1641=VECTOR('',#6532,10.) ;
#1642=VECTOR('',#6539,10.) ;
#1643=VECTOR('',#6542,10.) ;
#1644=VECTOR('',#6543,10.) ;
#1645=VECTOR('',#6544,10.) ;
#1646=VECTOR('',#6557,2.665) ;
#1647=VECTOR('',#6572,10.) ;
#1648=VECTOR('',#6573,10.) ;
#1649=VECTOR('',#6576,10.) ;
#1650=VECTOR('',#6579,10.) ;
#1651=VECTOR('',#6582,10.) ;
#1652=VECTOR('',#6585,10.) ;
#1653=VECTOR('',#6588,2.665) ;
#1654=VECTOR('',#6603,10.) ;
#1655=VECTOR('',#6612,10.) ;
#1656=VECTOR('',#6615,10.) ;
#1657=VECTOR('',#6616,10.) ;
#1658=VECTOR('',#6617,10.) ;
#1659=VECTOR('',#6620,10.) ;
#1660=VECTOR('',#6631,10.) ;
#1661=VECTOR('',#6632,10.) ;
#1662=VECTOR('',#6637,10.) ;
#1663=VECTOR('',#6656,10.) ;
#1664=VECTOR('',#6681,10.) ;
#1665=VECTOR('',#6684,10.) ;
#1666=VECTOR('',#6691,10.) ;
#1667=VECTOR('',#6696,10.) ;
#1668=VECTOR('',#6711,10.) ;
#1669=VECTOR('',#6712,10.) ;
#1670=VECTOR('',#6727,10.) ;
#1671=VECTOR('',#6728,10.) ;
#1672=VECTOR('',#6729,10.) ;
#1673=VECTOR('',#6732,10.) ;
#1674=VECTOR('',#6739,10.) ;
#1675=VECTOR('',#6744,10.) ;
#1676=VECTOR('',#6747,10.) ;
#1677=VECTOR('',#6750,10.) ;
#1678=VECTOR('',#6751,10.) ;
#1679=VECTOR('',#6754,10.) ;
#1680=VECTOR('',#6755,10.) ;
#1681=VECTOR('',#6768,10.) ;
#1682=VECTOR('',#6773,10.) ;
#1683=VECTOR('',#6776,10.) ;
#1684=VECTOR('',#6779,10.) ;
#1685=VECTOR('',#6780,10.) ;
#1686=VECTOR('',#6783,10.) ;
#1687=VECTOR('',#6788,10.) ;
#1688=VECTOR('',#6789,10.) ;
#1689=VECTOR('',#6792,10.) ;
#1690=VECTOR('',#6805,10.) ;
#1691=VECTOR('',#6806,10.) ;
#1692=VECTOR('',#6813,10.) ;
#1693=VECTOR('',#6814,10.) ;
#1694=VECTOR('',#6821,10.) ;
#1695=VECTOR('',#6822,10.) ;
#1696=VECTOR('',#6823,10.) ;
#1697=VECTOR('',#6826,10.) ;
#1698=VECTOR('',#6831,10.) ;
#1699=VECTOR('',#6832,10.) ;
#1700=VECTOR('',#6835,10.) ;
#1701=VECTOR('',#6840,10.) ;
#1702=VECTOR('',#6841,10.) ;
#1703=VECTOR('',#6844,10.) ;
#1704=VECTOR('',#6849,10.) ;
#1705=VECTOR('',#6850,10.) ;
#1706=VECTOR('',#6853,10.) ;
#1707=VECTOR('',#6858,10.) ;
#1708=VECTOR('',#6859,10.) ;
#1987=CIRCLE('',#5753,1.75) ;
#1988=CIRCLE('',#5754,1.75) ;
#1989=CIRCLE('',#5756,3.98) ;
#1990=CIRCLE('',#5757,3.98) ;
#1991=CIRCLE('',#5759,3.98) ;
#1992=CIRCLE('',#5760,3.98) ;
#1993=CIRCLE('',#5777,0.25) ;
#1994=CIRCLE('',#5778,2.665) ;
#1995=CIRCLE('',#5779,0.25) ;
#1996=CIRCLE('',#5780,2.915) ;
#1997=CIRCLE('',#5782,0.25) ;
#1998=CIRCLE('',#5784,0.249999999999999) ;
#1999=CIRCLE('',#5785,2.915) ;
#2000=CIRCLE('',#5786,2.665) ;
#2001=CIRCLE('',#5790,2.665) ;
#2002=CIRCLE('',#5792,16.3358074534161) ;
#2003=CIRCLE('',#5793,2.83595375255767) ;
#2004=CIRCLE('',#5794,2.915) ;
#2005=CIRCLE('',#5796,0.25) ;
#2006=CIRCLE('',#5797,2.665) ;
#2007=CIRCLE('',#5798,2.665) ;
#2008=CIRCLE('',#5800,2.665) ;
#2009=CIRCLE('',#5802,2.915) ;
#2010=CIRCLE('',#5803,0.25) ;
#2011=CIRCLE('',#5804,2.665) ;
#2012=CIRCLE('',#5805,2.665) ;
#2013=CIRCLE('',#5807,3.05499364382027) ;
#2014=CIRCLE('',#5808,16.3358074534161) ;
#2015=CIRCLE('',#5809,2.915) ;
#2016=CIRCLE('',#5810,2.915) ;
#2017=CIRCLE('',#5812,2.665) ;
#2018=CIRCLE('',#5814,0.25) ;
#2019=CIRCLE('',#5815,2.665) ;
#2020=CIRCLE('',#5816,0.25) ;
#2021=CIRCLE('',#5818,0.25) ;
#2022=CIRCLE('',#5820,0.249999999999999) ;
#2023=CIRCLE('',#5821,2.665) ;
#2024=CIRCLE('',#5825,2.665) ;
#2025=CIRCLE('',#5827,0.249999999999999) ;
#2026=CIRCLE('',#5829,0.249999999999999) ;
#2027=CIRCLE('',#5831,0.25) ;
#2028=CIRCLE('',#5832,0.249999999999999) ;
#2029=CIRCLE('',#5834,1.27) ;
#2030=CIRCLE('',#5835,1.52) ;
#2031=CIRCLE('',#5837,3.30499364382027) ;
#2032=CIRCLE('',#5839,3.08595375255767) ;
#2033=CIRCLE('',#5841,0.25) ;
#2034=CIRCLE('',#5842,0.25) ;
#2035=CIRCLE('',#5844,0.25) ;
#2036=CIRCLE('',#5845,16.5858074534161) ;
#2037=CIRCLE('',#5846,16.3358074534161) ;
#2038=CIRCLE('',#5848,0.25) ;
#2039=CIRCLE('',#5849,16.5858074534161) ;
#2040=CIRCLE('',#5851,16.5858074534161) ;
#2041=CIRCLE('',#5854,0.249999999999999) ;
#2042=CIRCLE('',#5856,0.25) ;
#2043=CIRCLE('',#5858,0.25) ;
#2044=CIRCLE('',#5859,0.249999999999999) ;
#2045=CIRCLE('',#5861,0.249999999999999) ;
#2046=CIRCLE('',#5862,1.27) ;
#2047=CIRCLE('',#5863,1.52) ;
#2048=CIRCLE('',#5865,0.249999999999999) ;
#2049=CIRCLE('',#5869,0.249999999999995) ;
#2050=CIRCLE('',#5871,0.249999999999995) ;
#2051=CIRCLE('',#5873,10.1848235398934) ;
#2052=CIRCLE('',#5881,10.1848235398934) ;
#2053=CIRCLE('',#5886,13.3598235398934) ;
#2054=CIRCLE('',#5893,13.3598235398934) ;
#2055=CIRCLE('',#5903,2.665) ;
#2056=CIRCLE('',#5906,2.665) ;
#2057=CIRCLE('',#5909,3.08595375255767) ;
#2058=CIRCLE('',#5912,16.5858074534161) ;
#2059=CIRCLE('',#5915,3.30499364382027) ;
#2060=CIRCLE('',#5918,0.249999999999995) ;
#2061=CIRCLE('',#5921,0.249999999999995) ;
#2269=VERTEX_POINT('',#8131) ;
#2270=VERTEX_POINT('',#8133) ;
#2271=VERTEX_POINT('',#8137) ;
#2272=VERTEX_POINT('',#8139) ;
#2273=VERTEX_POINT('',#8143) ;
#2274=VERTEX_POINT('',#8145) ;
#2275=VERTEX_POINT('',#8149) ;
#2276=VERTEX_POINT('',#8150) ;
#2277=VERTEX_POINT('',#8152) ;
#2278=VERTEX_POINT('',#8154) ;
#2279=VERTEX_POINT('',#8156) ;
#2280=VERTEX_POINT('',#8158) ;
#2281=VERTEX_POINT('',#8162) ;
#2282=VERTEX_POINT('',#8164) ;
#2283=VERTEX_POINT('',#8166) ;
#2284=VERTEX_POINT('',#8168) ;
#2285=VERTEX_POINT('',#8170) ;
#2286=VERTEX_POINT('',#8172) ;
#2287=VERTEX_POINT('',#8176) ;
#2288=VERTEX_POINT('',#8180) ;
#2289=VERTEX_POINT('',#8184) ;
#2290=VERTEX_POINT('',#8188) ;
#2291=VERTEX_POINT('',#8192) ;
#2292=VERTEX_POINT('',#8194) ;
#2293=VERTEX_POINT('',#8198) ;
#2294=VERTEX_POINT('',#8200) ;
#2295=VERTEX_POINT('',#8204) ;
#2296=VERTEX_POINT('',#8206) ;
#2297=VERTEX_POINT('',#8208) ;
#2298=VERTEX_POINT('',#8212) ;
#2299=VERTEX_POINT('',#8235) ;
#2300=VERTEX_POINT('',#8236) ;
#2301=VERTEX_POINT('',#8238) ;
#2302=VERTEX_POINT('',#8240) ;
#2303=VERTEX_POINT('',#8244) ;
#2304=VERTEX_POINT('',#8245) ;
#2305=VERTEX_POINT('',#8250) ;
#2306=VERTEX_POINT('',#8251) ;
#2307=VERTEX_POINT('',#8259) ;
#2308=VERTEX_POINT('',#8261) ;
#2309=VERTEX_POINT('',#8265) ;
#2310=VERTEX_POINT('',#8269) ;
#2311=VERTEX_POINT('',#8270) ;
#2312=VERTEX_POINT('',#8272) ;
#2313=VERTEX_POINT('',#8274) ;
#2314=VERTEX_POINT('',#8276) ;
#2315=VERTEX_POINT('',#8278) ;
#2316=VERTEX_POINT('',#8281) ;
#2317=VERTEX_POINT('',#8284) ;
#2318=VERTEX_POINT('',#8286) ;
#2319=VERTEX_POINT('',#8290) ;
#2320=VERTEX_POINT('',#8294) ;
#2321=VERTEX_POINT('',#8296) ;
#2322=VERTEX_POINT('',#8298) ;
#2323=VERTEX_POINT('',#8302) ;
#2324=VERTEX_POINT('',#8303) ;
#2325=VERTEX_POINT('',#8305) ;
#2326=VERTEX_POINT('',#8307) ;
#2327=VERTEX_POINT('',#8309) ;
#2328=VERTEX_POINT('',#8311) ;
#2329=VERTEX_POINT('',#8314) ;
#2330=VERTEX_POINT('',#8315) ;
#2331=VERTEX_POINT('',#8317) ;
#2332=VERTEX_POINT('',#8319) ;
#2333=VERTEX_POINT('',#8323) ;
#2334=VERTEX_POINT('',#8327) ;
#2335=VERTEX_POINT('',#8329) ;
#2336=VERTEX_POINT('',#8333) ;
#2337=VERTEX_POINT('',#8337) ;
#2338=VERTEX_POINT('',#8343) ;
#2339=VERTEX_POINT('',#8345) ;
#2340=VERTEX_POINT('',#8349) ;
#2341=VERTEX_POINT('',#8377) ;
#2342=VERTEX_POINT('',#8381) ;
#2343=VERTEX_POINT('',#8382) ;
#2344=VERTEX_POINT('',#8387) ;
#2345=VERTEX_POINT('',#8389) ;
#2346=VERTEX_POINT('',#8396) ;
#2347=VERTEX_POINT('',#8397) ;
#2348=VERTEX_POINT('',#8440) ;
#2349=VERTEX_POINT('',#8469) ;
#2350=VERTEX_POINT('',#8484) ;
#2351=VERTEX_POINT('',#8518) ;
#2352=VERTEX_POINT('',#8523) ;
#2353=VERTEX_POINT('',#8525) ;
#2354=VERTEX_POINT('',#8530) ;
#2355=VERTEX_POINT('',#8586) ;
#2356=VERTEX_POINT('',#8587) ;
#2357=VERTEX_POINT('',#8592) ;
#2358=VERTEX_POINT('',#8594) ;
#2359=VERTEX_POINT('',#8631) ;
#2360=VERTEX_POINT('',#8632) ;
#2361=VERTEX_POINT('',#8665) ;
#2362=VERTEX_POINT('',#8692) ;
#2363=VERTEX_POINT('',#8702) ;
#2364=VERTEX_POINT('',#8719) ;
#2365=VERTEX_POINT('',#8723) ;
#2366=VERTEX_POINT('',#8727) ;
#2367=VERTEX_POINT('',#8729) ;
#2368=VERTEX_POINT('',#8733) ;
#2369=VERTEX_POINT('',#8734) ;
#2370=VERTEX_POINT('',#8739) ;
#2371=VERTEX_POINT('',#8740) ;
#2372=VERTEX_POINT('',#8769) ;
#2373=VERTEX_POINT('',#8770) ;
#2374=VERTEX_POINT('',#8798) ;
#2375=VERTEX_POINT('',#8800) ;
#2376=VERTEX_POINT('',#8802) ;
#2377=VERTEX_POINT('',#8804) ;
#2378=VERTEX_POINT('',#8812) ;
#2379=VERTEX_POINT('',#8818) ;
#2380=VERTEX_POINT('',#8820) ;
#2381=VERTEX_POINT('',#8822) ;
#2382=VERTEX_POINT('',#8824) ;
#2383=VERTEX_POINT('',#8831) ;
#2384=VERTEX_POINT('',#8832) ;
#2385=VERTEX_POINT('',#8904) ;
#2386=VERTEX_POINT('',#8906) ;
#2387=VERTEX_POINT('',#8933) ;
#2388=VERTEX_POINT('',#8937) ;
#2389=VERTEX_POINT('',#8941) ;
#2390=VERTEX_POINT('',#8945) ;
#2391=VERTEX_POINT('',#9042) ;
#2392=VERTEX_POINT('',#9048) ;
#2393=VERTEX_POINT('',#9054) ;
#2394=VERTEX_POINT('',#9056) ;
#2395=VERTEX_POINT('',#9060) ;
#2396=VERTEX_POINT('',#9064) ;
#2397=VERTEX_POINT('',#9068) ;
#2398=VERTEX_POINT('',#9072) ;
#2399=VERTEX_POINT('',#9076) ;
#2400=VERTEX_POINT('',#9080) ;
#2401=VERTEX_POINT('',#9084) ;
#2402=VERTEX_POINT('',#9088) ;
#2746=EDGE_CURVE('',#2269,#2269,#1987,.T.) ;
#2747=EDGE_CURVE('',#2269,#2270,#1221,.T.) ;
#2748=EDGE_CURVE('',#2270,#2270,#1988,.T.) ;
#2749=EDGE_CURVE('',#2271,#2271,#1989,.T.) ;
#2750=EDGE_CURVE('',#2271,#2272,#1222,.T.) ;
#2751=EDGE_CURVE('',#2272,#2272,#1990,.T.) ;
#2752=EDGE_CURVE('',#2273,#2273,#1991,.T.) ;
#2753=EDGE_CURVE('',#2273,#2274,#1223,.T.) ;
#2754=EDGE_CURVE('',#2274,#2274,#1992,.T.) ;
#2755=EDGE_CURVE('',#2275,#2276,#378,.T.) ;
#2756=EDGE_CURVE('',#2277,#2275,#1224,.T.) ;
#2757=EDGE_CURVE('',#2277,#2278,#1225,.T.) ;
#2758=EDGE_CURVE('',#2278,#2279,#1226,.T.) ;
#2759=EDGE_CURVE('',#2280,#2279,#379,.T.) ;
#2760=EDGE_CURVE('',#2276,#2280,#1227,.T.) ;
#2761=EDGE_CURVE('',#2279,#2281,#1228,.T.) ;
#2762=EDGE_CURVE('',#2282,#2278,#1229,.T.) ;
#2763=EDGE_CURVE('',#2283,#2282,#1230,.T.) ;
#2764=EDGE_CURVE('',#2284,#2283,#1231,.T.) ;
#2765=EDGE_CURVE('',#2285,#2284,#1232,.T.) ;
#2766=EDGE_CURVE('',#2286,#2285,#1233,.T.) ;
#2767=EDGE_CURVE('',#2281,#2286,#1234,.T.) ;
#2768=EDGE_CURVE('',#2287,#2277,#1235,.T.) ;
#2769=EDGE_CURVE('',#2287,#2282,#1236,.T.) ;
#2770=EDGE_CURVE('',#2288,#2287,#1237,.T.) ;
#2771=EDGE_CURVE('',#2288,#2283,#1238,.T.) ;
#2772=EDGE_CURVE('',#2289,#2288,#1239,.T.) ;
#2773=EDGE_CURVE('',#2289,#2284,#1240,.T.) ;
#2774=EDGE_CURVE('',#2285,#2290,#1241,.T.) ;
#2775=EDGE_CURVE('',#2290,#2289,#1242,.T.) ;
#2776=EDGE_CURVE('',#2291,#2275,#1243,.T.) ;
#2777=EDGE_CURVE('',#2292,#2291,#1244,.T.) ;
#2778=EDGE_CURVE('',#2290,#2292,#1245,.T.) ;
#2779=EDGE_CURVE('',#2293,#2280,#1246,.T.) ;
#2780=EDGE_CURVE('',#2294,#2293,#1247,.T.) ;
#2781=EDGE_CURVE('',#2276,#2294,#1248,.T.) ;
#2782=EDGE_CURVE('',#2281,#2295,#380,.T.) ;
#2783=EDGE_CURVE('',#2296,#2295,#381,.T.) ;
#2784=EDGE_CURVE('',#2296,#2297,#1249,.T.) ;
#2785=EDGE_CURVE('',#2297,#2293,#382,.T.) ;
#2786=EDGE_CURVE('',#2286,#2298,#1250,.T.) ;
#2787=EDGE_CURVE('',#2295,#2298,#238,.T.) ;
#2788=EDGE_CURVE('',#2299,#2300,#1993,.T.) ;
#2789=EDGE_CURVE('',#2300,#2301,#1994,.T.) ;
#2790=EDGE_CURVE('',#2301,#2302,#1995,.T.) ;
#2791=EDGE_CURVE('',#2302,#2299,#1996,.T.) ;
#2792=EDGE_CURVE('',#2303,#2304,#1997,.T.) ;
#2793=EDGE_CURVE('',#2304,#2302,#1251,.T.) ;
#2794=EDGE_CURVE('',#2301,#2303,#1252,.T.) ;
#2795=EDGE_CURVE('',#2305,#2306,#1998,.T.) ;
#2796=EDGE_CURVE('',#2306,#2304,#1999,.T.) ;
#2797=EDGE_CURVE('',#2303,#2305,#2000,.T.) ;
#2798=EDGE_CURVE('',#2299,#2306,#1253,.T.) ;
#2799=EDGE_CURVE('',#2305,#2300,#1254,.T.) ;
#2800=EDGE_CURVE('',#2307,#2301,#1255,.T.) ;
#2801=EDGE_CURVE('',#2307,#2308,#1256,.T.) ;
#2802=EDGE_CURVE('',#2308,#2303,#1257,.T.) ;
#2803=EDGE_CURVE('',#2309,#2300,#1258,.T.) ;
#2804=EDGE_CURVE('',#2309,#2307,#2001,.T.) ;
#2805=EDGE_CURVE('',#2310,#2311,#2002,.T.) ;
#2806=EDGE_CURVE('',#2312,#2310,#1259,.T.) ;
#2807=EDGE_CURVE('',#2313,#2312,#2003,.T.) ;
#2808=EDGE_CURVE('',#2314,#2313,#1260,.T.) ;
#2809=EDGE_CURVE('',#2315,#2314,#1261,.T.) ;
#2810=EDGE_CURVE('',#2311,#2315,#1262,.T.) ;
#2811=EDGE_CURVE('',#2316,#2316,#2004,.T.) ;
#2812=EDGE_CURVE('',#2316,#2317,#2005,.T.) ;
#2813=EDGE_CURVE('',#2317,#2318,#2006,.T.) ;
#2814=EDGE_CURVE('',#2318,#2317,#2007,.T.) ;
#2815=EDGE_CURVE('',#2318,#2319,#1263,.T.) ;
#2816=EDGE_CURVE('',#2319,#2319,#2008,.T.) ;
#2817=EDGE_CURVE('',#2320,#2320,#2009,.T.) ;
#2818=EDGE_CURVE('',#2320,#2321,#2010,.T.) ;
#2819=EDGE_CURVE('',#2321,#2322,#2011,.T.) ;
#2820=EDGE_CURVE('',#2322,#2321,#2012,.T.) ;
#2821=EDGE_CURVE('',#2323,#2324,#1264,.T.) ;
#2822=EDGE_CURVE('',#2325,#2323,#1265,.T.) ;
#2823=EDGE_CURVE('',#2326,#2325,#2013,.T.) ;
#2824=EDGE_CURVE('',#2327,#2326,#1266,.T.) ;
#2825=EDGE_CURVE('',#2328,#2327,#2014,.T.) ;
#2826=EDGE_CURVE('',#2324,#2328,#1267,.T.) ;
#2827=EDGE_CURVE('',#2329,#2330,#2015,.T.) ;
#2828=EDGE_CURVE('',#2331,#2329,#1268,.T.) ;
#2829=EDGE_CURVE('',#2332,#2331,#2016,.T.) ;
#2830=EDGE_CURVE('',#2330,#2332,#1269,.T.) ;
#2831=EDGE_CURVE('',#2322,#2333,#1270,.T.) ;
#2832=EDGE_CURVE('',#2333,#2333,#2017,.T.) ;
#2833=EDGE_CURVE('',#2330,#2334,#2018,.T.) ;
#2834=EDGE_CURVE('',#2334,#2335,#2019,.T.) ;
#2835=EDGE_CURVE('',#2335,#2329,#2020,.T.) ;
#2836=EDGE_CURVE('',#2336,#2331,#2021,.T.) ;
#2837=EDGE_CURVE('',#2335,#2336,#1271,.T.) ;
#2838=EDGE_CURVE('',#2337,#2332,#2022,.T.) ;
#2839=EDGE_CURVE('',#2336,#2337,#2023,.T.) ;
#2840=EDGE_CURVE('',#2337,#2334,#1272,.T.) ;
#2841=EDGE_CURVE('',#2338,#2335,#1273,.T.) ;
#2842=EDGE_CURVE('',#2338,#2339,#1274,.T.) ;
#2843=EDGE_CURVE('',#2339,#2336,#1275,.T.) ;
#2844=EDGE_CURVE('',#2340,#2334,#1276,.T.) ;
#2845=EDGE_CURVE('',#2340,#2338,#2024,.T.) ;
#2846=EDGE_CURVE('',#2298,#2341,#383,.T.) ;
#2847=EDGE_CURVE('',#2341,#2296,#2025,.T.) ;
#2848=EDGE_CURVE('',#2342,#2343,#2026,.T.) ;
#2849=EDGE_CURVE('',#2343,#2296,#1277,.T.) ;
#2850=EDGE_CURVE('',#2341,#2342,#1278,.T.) ;
#2851=EDGE_CURVE('',#2324,#2344,#2027,.T.) ;
#2852=EDGE_CURVE('',#2344,#2345,#1279,.T.) ;
#2853=EDGE_CURVE('',#2345,#2323,#2028,.T.) ;
#2854=EDGE_CURVE('',#2324,#2343,#2029,.T.) ;
#2855=EDGE_CURVE('',#2342,#2344,#2030,.T.) ;
#2856=EDGE_CURVE('',#2346,#2347,#2031,.T.) ;
#2857=EDGE_CURVE('',#2347,#2326,#239,.T.) ;
#2858=EDGE_CURVE('',#2325,#2346,#240,.T.) ;
#2859=EDGE_CURVE('',#2348,#2313,#241,.T.) ;
#2860=EDGE_CURVE('',#2312,#2349,#242,.T.) ;
#2861=EDGE_CURVE('',#2349,#2348,#2032,.T.) ;
#2862=EDGE_CURVE('',#2310,#2350,#243,.T.) ;
#2863=EDGE_CURVE('',#2350,#2349,#1280,.T.) ;
#2864=EDGE_CURVE('',#2351,#2328,#244,.T.) ;
#2865=EDGE_CURVE('',#2328,#2352,#2033,.T.) ;
#2866=EDGE_CURVE('',#2352,#2353,#245,.T.) ;
#2867=EDGE_CURVE('',#2353,#2354,#246,.T.) ;
#2868=EDGE_CURVE('',#2354,#2351,#247,.T.) ;
#2869=EDGE_CURVE('',#2355,#2356,#248,.T.) ;
#2870=EDGE_CURVE('',#2356,#2357,#2034,.T.) ;
#2871=EDGE_CURVE('',#2357,#2358,#249,.T.) ;
#2872=EDGE_CURVE('',#2358,#2355,#250,.T.) ;
#2873=EDGE_CURVE('',#2359,#2360,#2035,.T.) ;
#2874=EDGE_CURVE('',#2360,#2357,#2036,.T.) ;
#2875=EDGE_CURVE('',#2356,#2359,#2037,.T.) ;
#2876=EDGE_CURVE('',#2353,#2360,#251,.T.) ;
#2877=EDGE_CURVE('',#2359,#2354,#252,.T.) ;
#2878=EDGE_CURVE('',#2311,#2361,#2038,.T.) ;
#2879=EDGE_CURVE('',#2361,#2350,#2039,.T.) ;
#2880=EDGE_CURVE('',#2358,#2361,#253,.T.) ;
#2881=EDGE_CURVE('',#2311,#2362,#254,.T.) ;
#2882=EDGE_CURVE('',#2362,#2355,#255,.T.) ;
#2883=EDGE_CURVE('',#2363,#2352,#2040,.T.) ;
#2884=EDGE_CURVE('',#2327,#2363,#256,.T.) ;
#2885=EDGE_CURVE('',#2347,#2363,#1281,.T.) ;
#2886=EDGE_CURVE('',#2348,#2364,#1282,.T.) ;
#2887=EDGE_CURVE('',#2364,#2314,#2041,.T.) ;
#2888=EDGE_CURVE('',#2323,#2365,#2042,.T.) ;
#2889=EDGE_CURVE('',#2365,#2346,#1283,.T.) ;
#2890=EDGE_CURVE('',#2314,#2366,#2043,.T.) ;
#2891=EDGE_CURVE('',#2366,#2367,#1284,.T.) ;
#2892=EDGE_CURVE('',#2367,#2315,#2044,.T.) ;
#2893=EDGE_CURVE('',#2368,#2369,#2045,.T.) ;
#2894=EDGE_CURVE('',#2369,#2315,#2046,.T.) ;
#2895=EDGE_CURVE('',#2367,#2368,#2047,.T.) ;
#2896=EDGE_CURVE('',#2370,#2371,#2048,.T.) ;
#2897=EDGE_CURVE('',#2371,#2369,#1285,.T.) ;
#2898=EDGE_CURVE('',#2368,#2370,#1286,.T.) ;
#2899=EDGE_CURVE('',#2372,#2373,#257,.T.) ;
#2900=EDGE_CURVE('',#2373,#2371,#384,.T.) ;
#2901=EDGE_CURVE('',#2370,#2372,#385,.T.) ;
#2902=EDGE_CURVE('',#2364,#2366,#2049,.T.) ;
#2903=EDGE_CURVE('',#2345,#2365,#2050,.T.) ;
#2904=EDGE_CURVE('',#2374,#2343,#1287,.T.) ;
#2905=EDGE_CURVE('',#2374,#2375,#1288,.T.) ;
#2906=EDGE_CURVE('',#2376,#2375,#1289,.T.) ;
#2907=EDGE_CURVE('',#2377,#2376,#2051,.T.) ;
#2908=EDGE_CURVE('',#2297,#2377,#1290,.T.) ;
#2909=EDGE_CURVE('',#2374,#2351,#386,.T.) ;
#2910=EDGE_CURVE('',#2359,#2356,#1291,.T.) ;
#2911=EDGE_CURVE('',#2362,#2378,#387,.T.) ;
#2912=EDGE_CURVE('',#2378,#2374,#1292,.T.) ;
#2913=EDGE_CURVE('',#2369,#2378,#1293,.T.) ;
#2914=EDGE_CURVE('',#2379,#2371,#1294,.T.) ;
#2915=EDGE_CURVE('',#2380,#2379,#1295,.T.) ;
#2916=EDGE_CURVE('',#2381,#2380,#2052,.T.) ;
#2917=EDGE_CURVE('',#2382,#2381,#1296,.T.) ;
#2918=EDGE_CURVE('',#2378,#2382,#1297,.T.) ;
#2919=EDGE_CURVE('',#2379,#2294,#388,.T.) ;
#2920=EDGE_CURVE('',#2373,#2291,#389,.T.) ;
#2921=EDGE_CURVE('',#2383,#2384,#2053,.T.) ;
#2922=EDGE_CURVE('',#2384,#2377,#258,.T.) ;
#2923=EDGE_CURVE('',#2376,#2383,#259,.T.) ;
#2924=EDGE_CURVE('',#2384,#2293,#1298,.T.) ;
#2925=EDGE_CURVE('',#2375,#2385,#390,.T.) ;
#2926=EDGE_CURVE('',#2385,#2386,#260,.T.) ;
#2927=EDGE_CURVE('',#2386,#2383,#1299,.T.) ;
#2928=EDGE_CURVE('',#2372,#2292,#1300,.T.) ;
#2929=EDGE_CURVE('',#2387,#2384,#1301,.T.) ;
#2930=EDGE_CURVE('',#2294,#2387,#1302,.T.) ;
#2931=EDGE_CURVE('',#2388,#2383,#1303,.T.) ;
#2932=EDGE_CURVE('',#2387,#2388,#2054,.T.) ;
#2933=EDGE_CURVE('',#2389,#2386,#1304,.T.) ;
#2934=EDGE_CURVE('',#2388,#2389,#1305,.T.) ;
#2935=EDGE_CURVE('',#2390,#2385,#1306,.T.) ;
#2936=EDGE_CURVE('',#2389,#2390,#261,.T.) ;
#2937=EDGE_CURVE('',#2390,#2382,#391,.T.) ;
#2938=EDGE_CURVE('',#2381,#2388,#262,.T.) ;
#2939=EDGE_CURVE('',#2387,#2380,#263,.T.) ;
#2940=EDGE_CURVE('',#2391,#2305,#1307,.T.) ;
#2941=EDGE_CURVE('',#2391,#2309,#1308,.T.) ;
#2942=EDGE_CURVE('',#2308,#2391,#2055,.T.) ;
#2943=EDGE_CURVE('',#2392,#2337,#1309,.T.) ;
#2944=EDGE_CURVE('',#2392,#2340,#1310,.T.) ;
#2945=EDGE_CURVE('',#2339,#2392,#2056,.T.) ;
#2946=EDGE_CURVE('',#2393,#2348,#1311,.T.) ;
#2947=EDGE_CURVE('',#2394,#2393,#1312,.T.) ;
#2948=EDGE_CURVE('',#2394,#2364,#1313,.T.) ;
#2949=EDGE_CURVE('',#2395,#2349,#1314,.T.) ;
#2950=EDGE_CURVE('',#2395,#2393,#2057,.T.) ;
#2951=EDGE_CURVE('',#2396,#2350,#1315,.T.) ;
#2952=EDGE_CURVE('',#2395,#2396,#1316,.T.) ;
#2953=EDGE_CURVE('',#2397,#2363,#1317,.T.) ;
#2954=EDGE_CURVE('',#2397,#2396,#2058,.T.) ;
#2955=EDGE_CURVE('',#2398,#2347,#1318,.T.) ;
#2956=EDGE_CURVE('',#2397,#2398,#1319,.T.) ;
#2957=EDGE_CURVE('',#2399,#2346,#1320,.T.) ;
#2958=EDGE_CURVE('',#2399,#2398,#2059,.T.) ;
#2959=EDGE_CURVE('',#2400,#2365,#1321,.T.) ;
#2960=EDGE_CURVE('',#2399,#2400,#1322,.T.) ;
#2961=EDGE_CURVE('',#2401,#2345,#1323,.T.) ;
#2962=EDGE_CURVE('',#2401,#2400,#2060,.T.) ;
#2963=EDGE_CURVE('',#2402,#2366,#1324,.T.) ;
#2964=EDGE_CURVE('',#2401,#2402,#1325,.T.) ;
#2965=EDGE_CURVE('',#2394,#2402,#2061,.T.) ;
#3528=ORIENTED_EDGE('',*,*,#2746,.F.) ;
#3529=ORIENTED_EDGE('',*,*,#2747,.T.) ;
#3530=ORIENTED_EDGE('',*,*,#2748,.F.) ;
#3531=ORIENTED_EDGE('',*,*,#2747,.F.) ;
#3532=ORIENTED_EDGE('',*,*,#2749,.F.) ;
#3533=ORIENTED_EDGE('',*,*,#2750,.T.) ;
#3534=ORIENTED_EDGE('',*,*,#2751,.F.) ;
#3535=ORIENTED_EDGE('',*,*,#2750,.F.) ;
#3536=ORIENTED_EDGE('',*,*,#2752,.F.) ;
#3537=ORIENTED_EDGE('',*,*,#2753,.T.) ;
#3538=ORIENTED_EDGE('',*,*,#2754,.F.) ;
#3539=ORIENTED_EDGE('',*,*,#2753,.F.) ;
#3540=ORIENTED_EDGE('',*,*,#2755,.F.) ;
#3541=ORIENTED_EDGE('',*,*,#2756,.F.) ;
#3542=ORIENTED_EDGE('',*,*,#2757,.T.) ;
#3543=ORIENTED_EDGE('',*,*,#2758,.T.) ;
#3544=ORIENTED_EDGE('',*,*,#2759,.F.) ;
#3545=ORIENTED_EDGE('',*,*,#2760,.F.) ;
#3546=ORIENTED_EDGE('',*,*,#2761,.F.) ;
#3547=ORIENTED_EDGE('',*,*,#2758,.F.) ;
#3548=ORIENTED_EDGE('',*,*,#2762,.F.) ;
#3549=ORIENTED_EDGE('',*,*,#2763,.F.) ;
#3550=ORIENTED_EDGE('',*,*,#2764,.F.) ;
#3551=ORIENTED_EDGE('',*,*,#2765,.F.) ;
#3552=ORIENTED_EDGE('',*,*,#2766,.F.) ;
#3553=ORIENTED_EDGE('',*,*,#2767,.F.) ;
#3554=ORIENTED_EDGE('',*,*,#2752,.T.) ;
#3555=ORIENTED_EDGE('',*,*,#2768,.F.) ;
#3556=ORIENTED_EDGE('',*,*,#2769,.T.) ;
#3557=ORIENTED_EDGE('',*,*,#2762,.T.) ;
#3558=ORIENTED_EDGE('',*,*,#2757,.F.) ;
#3559=ORIENTED_EDGE('',*,*,#2770,.F.) ;
#3560=ORIENTED_EDGE('',*,*,#2771,.T.) ;
#3561=ORIENTED_EDGE('',*,*,#2763,.T.) ;
#3562=ORIENTED_EDGE('',*,*,#2769,.F.) ;
#3563=ORIENTED_EDGE('',*,*,#2772,.F.) ;
#3564=ORIENTED_EDGE('',*,*,#2773,.T.) ;
#3565=ORIENTED_EDGE('',*,*,#2764,.T.) ;
#3566=ORIENTED_EDGE('',*,*,#2771,.F.) ;
#3567=ORIENTED_EDGE('',*,*,#2748,.T.) ;
#3568=ORIENTED_EDGE('',*,*,#2774,.F.) ;
#3569=ORIENTED_EDGE('',*,*,#2765,.T.) ;
#3570=ORIENTED_EDGE('',*,*,#2773,.F.) ;
#3571=ORIENTED_EDGE('',*,*,#2775,.F.) ;
#3572=ORIENTED_EDGE('',*,*,#2776,.F.) ;
#3573=ORIENTED_EDGE('',*,*,#2777,.F.) ;
#3574=ORIENTED_EDGE('',*,*,#2778,.F.) ;
#3575=ORIENTED_EDGE('',*,*,#2775,.T.) ;
#3576=ORIENTED_EDGE('',*,*,#2772,.T.) ;
#3577=ORIENTED_EDGE('',*,*,#2770,.T.) ;
#3578=ORIENTED_EDGE('',*,*,#2768,.T.) ;
#3579=ORIENTED_EDGE('',*,*,#2756,.T.) ;
#3580=ORIENTED_EDGE('',*,*,#2751,.T.) ;
#3581=ORIENTED_EDGE('',*,*,#2760,.T.) ;
#3582=ORIENTED_EDGE('',*,*,#2779,.F.) ;
#3583=ORIENTED_EDGE('',*,*,#2780,.F.) ;
#3584=ORIENTED_EDGE('',*,*,#2781,.F.) ;
#3585=ORIENTED_EDGE('',*,*,#2759,.T.) ;
#3586=ORIENTED_EDGE('',*,*,#2761,.T.) ;
#3587=ORIENTED_EDGE('',*,*,#2782,.T.) ;
#3588=ORIENTED_EDGE('',*,*,#2783,.F.) ;
#3589=ORIENTED_EDGE('',*,*,#2784,.T.) ;
#3590=ORIENTED_EDGE('',*,*,#2785,.T.) ;
#3591=ORIENTED_EDGE('',*,*,#2779,.T.) ;
#3592=ORIENTED_EDGE('',*,*,#2767,.T.) ;
#3593=ORIENTED_EDGE('',*,*,#2786,.T.) ;
#3594=ORIENTED_EDGE('',*,*,#2787,.F.) ;
#3595=ORIENTED_EDGE('',*,*,#2782,.F.) ;
#3596=ORIENTED_EDGE('',*,*,#2788,.T.) ;
#3597=ORIENTED_EDGE('',*,*,#2789,.T.) ;
#3598=ORIENTED_EDGE('',*,*,#2790,.T.) ;
#3599=ORIENTED_EDGE('',*,*,#2791,.T.) ;
#3600=ORIENTED_EDGE('',*,*,#2792,.T.) ;
#3601=ORIENTED_EDGE('',*,*,#2793,.T.) ;
#3602=ORIENTED_EDGE('',*,*,#2790,.F.) ;
#3603=ORIENTED_EDGE('',*,*,#2794,.T.) ;
#3604=ORIENTED_EDGE('',*,*,#2795,.T.) ;
#3605=ORIENTED_EDGE('',*,*,#2796,.T.) ;
#3606=ORIENTED_EDGE('',*,*,#2792,.F.) ;
#3607=ORIENTED_EDGE('',*,*,#2797,.T.) ;
#3608=ORIENTED_EDGE('',*,*,#2788,.F.) ;
#3609=ORIENTED_EDGE('',*,*,#2798,.T.) ;
#3610=ORIENTED_EDGE('',*,*,#2795,.F.) ;
#3611=ORIENTED_EDGE('',*,*,#2799,.T.) ;
#3612=ORIENTED_EDGE('',*,*,#2794,.F.) ;
#3613=ORIENTED_EDGE('',*,*,#2800,.F.) ;
#3614=ORIENTED_EDGE('',*,*,#2801,.T.) ;
#3615=ORIENTED_EDGE('',*,*,#2802,.T.) ;
#3616=ORIENTED_EDGE('',*,*,#2789,.F.) ;
#3617=ORIENTED_EDGE('',*,*,#2803,.F.) ;
#3618=ORIENTED_EDGE('',*,*,#2804,.T.) ;
#3619=ORIENTED_EDGE('',*,*,#2800,.T.) ;
#3620=ORIENTED_EDGE('',*,*,#2805,.F.) ;
#3621=ORIENTED_EDGE('',*,*,#2806,.F.) ;
#3622=ORIENTED_EDGE('',*,*,#2807,.F.) ;
#3623=ORIENTED_EDGE('',*,*,#2808,.F.) ;
#3624=ORIENTED_EDGE('',*,*,#2809,.F.) ;
#3625=ORIENTED_EDGE('',*,*,#2810,.F.) ;
#3626=ORIENTED_EDGE('',*,*,#2811,.F.) ;
#3627=ORIENTED_EDGE('',*,*,#2791,.F.) ;
#3628=ORIENTED_EDGE('',*,*,#2793,.F.) ;
#3629=ORIENTED_EDGE('',*,*,#2796,.F.) ;
#3630=ORIENTED_EDGE('',*,*,#2798,.F.) ;
#3631=ORIENTED_EDGE('',*,*,#2811,.T.) ;
#3632=ORIENTED_EDGE('',*,*,#2812,.T.) ;
#3633=ORIENTED_EDGE('',*,*,#2813,.T.) ;
#3634=ORIENTED_EDGE('',*,*,#2814,.T.) ;
#3635=ORIENTED_EDGE('',*,*,#2812,.F.) ;
#3636=ORIENTED_EDGE('',*,*,#2814,.F.) ;
#3637=ORIENTED_EDGE('',*,*,#2815,.T.) ;
#3638=ORIENTED_EDGE('',*,*,#2816,.T.) ;
#3639=ORIENTED_EDGE('',*,*,#2815,.F.) ;
#3640=ORIENTED_EDGE('',*,*,#2813,.F.) ;
#3641=ORIENTED_EDGE('',*,*,#2817,.T.) ;
#3642=ORIENTED_EDGE('',*,*,#2818,.T.) ;
#3643=ORIENTED_EDGE('',*,*,#2819,.T.) ;
#3644=ORIENTED_EDGE('',*,*,#2820,.T.) ;
#3645=ORIENTED_EDGE('',*,*,#2818,.F.) ;
#3646=ORIENTED_EDGE('',*,*,#2821,.F.) ;
#3647=ORIENTED_EDGE('',*,*,#2822,.F.) ;
#3648=ORIENTED_EDGE('',*,*,#2823,.F.) ;
#3649=ORIENTED_EDGE('',*,*,#2824,.F.) ;
#3650=ORIENTED_EDGE('',*,*,#2825,.F.) ;
#3651=ORIENTED_EDGE('',*,*,#2826,.F.) ;
#3652=ORIENTED_EDGE('',*,*,#2827,.F.) ;
#3653=ORIENTED_EDGE('',*,*,#2828,.F.) ;
#3654=ORIENTED_EDGE('',*,*,#2829,.F.) ;
#3655=ORIENTED_EDGE('',*,*,#2830,.F.) ;
#3656=ORIENTED_EDGE('',*,*,#2817,.F.) ;
#3657=ORIENTED_EDGE('',*,*,#2820,.F.) ;
#3658=ORIENTED_EDGE('',*,*,#2831,.T.) ;
#3659=ORIENTED_EDGE('',*,*,#2832,.T.) ;
#3660=ORIENTED_EDGE('',*,*,#2831,.F.) ;
#3661=ORIENTED_EDGE('',*,*,#2819,.F.) ;
#3662=ORIENTED_EDGE('',*,*,#2833,.T.) ;
#3663=ORIENTED_EDGE('',*,*,#2834,.T.) ;
#3664=ORIENTED_EDGE('',*,*,#2835,.T.) ;
#3665=ORIENTED_EDGE('',*,*,#2827,.T.) ;
#3666=ORIENTED_EDGE('',*,*,#2836,.T.) ;
#3667=ORIENTED_EDGE('',*,*,#2828,.T.) ;
#3668=ORIENTED_EDGE('',*,*,#2835,.F.) ;
#3669=ORIENTED_EDGE('',*,*,#2837,.T.) ;
#3670=ORIENTED_EDGE('',*,*,#2838,.T.) ;
#3671=ORIENTED_EDGE('',*,*,#2829,.T.) ;
#3672=ORIENTED_EDGE('',*,*,#2836,.F.) ;
#3673=ORIENTED_EDGE('',*,*,#2839,.T.) ;
#3674=ORIENTED_EDGE('',*,*,#2833,.F.) ;
#3675=ORIENTED_EDGE('',*,*,#2830,.T.) ;
#3676=ORIENTED_EDGE('',*,*,#2838,.F.) ;
#3677=ORIENTED_EDGE('',*,*,#2840,.T.) ;
#3678=ORIENTED_EDGE('',*,*,#2837,.F.) ;
#3679=ORIENTED_EDGE('',*,*,#2841,.F.) ;
#3680=ORIENTED_EDGE('',*,*,#2842,.T.) ;
#3681=ORIENTED_EDGE('',*,*,#2843,.T.) ;
#3682=ORIENTED_EDGE('',*,*,#2834,.F.) ;
#3683=ORIENTED_EDGE('',*,*,#2844,.F.) ;
#3684=ORIENTED_EDGE('',*,*,#2845,.T.) ;
#3685=ORIENTED_EDGE('',*,*,#2841,.T.) ;
#3686=ORIENTED_EDGE('',*,*,#2787,.T.) ;
#3687=ORIENTED_EDGE('',*,*,#2846,.T.) ;
#3688=ORIENTED_EDGE('',*,*,#2847,.T.) ;
#3689=ORIENTED_EDGE('',*,*,#2783,.T.) ;
#3690=ORIENTED_EDGE('',*,*,#2848,.T.) ;
#3691=ORIENTED_EDGE('',*,*,#2849,.T.) ;
#3692=ORIENTED_EDGE('',*,*,#2847,.F.) ;
#3693=ORIENTED_EDGE('',*,*,#2850,.T.) ;
#3694=ORIENTED_EDGE('',*,*,#2851,.T.) ;
#3695=ORIENTED_EDGE('',*,*,#2852,.T.) ;
#3696=ORIENTED_EDGE('',*,*,#2853,.T.) ;
#3697=ORIENTED_EDGE('',*,*,#2821,.T.) ;
#3698=ORIENTED_EDGE('',*,*,#2851,.F.) ;
#3699=ORIENTED_EDGE('',*,*,#2854,.T.) ;
#3700=ORIENTED_EDGE('',*,*,#2848,.F.) ;
#3701=ORIENTED_EDGE('',*,*,#2855,.T.) ;
#3702=ORIENTED_EDGE('',*,*,#2856,.T.) ;
#3703=ORIENTED_EDGE('',*,*,#2857,.T.) ;
#3704=ORIENTED_EDGE('',*,*,#2823,.T.) ;
#3705=ORIENTED_EDGE('',*,*,#2858,.T.) ;
#3706=ORIENTED_EDGE('',*,*,#2859,.T.) ;
#3707=ORIENTED_EDGE('',*,*,#2807,.T.) ;
#3708=ORIENTED_EDGE('',*,*,#2860,.T.) ;
#3709=ORIENTED_EDGE('',*,*,#2861,.T.) ;
#3710=ORIENTED_EDGE('',*,*,#2806,.T.) ;
#3711=ORIENTED_EDGE('',*,*,#2862,.T.) ;
#3712=ORIENTED_EDGE('',*,*,#2863,.T.) ;
#3713=ORIENTED_EDGE('',*,*,#2860,.F.) ;
#3714=ORIENTED_EDGE('',*,*,#2864,.T.) ;
#3715=ORIENTED_EDGE('',*,*,#2865,.T.) ;
#3716=ORIENTED_EDGE('',*,*,#2866,.T.) ;
#3717=ORIENTED_EDGE('',*,*,#2867,.T.) ;
#3718=ORIENTED_EDGE('',*,*,#2868,.T.) ;
#3719=ORIENTED_EDGE('',*,*,#2869,.T.) ;
#3720=ORIENTED_EDGE('',*,*,#2870,.T.) ;
#3721=ORIENTED_EDGE('',*,*,#2871,.T.) ;
#3722=ORIENTED_EDGE('',*,*,#2872,.T.) ;
#3723=ORIENTED_EDGE('',*,*,#2873,.T.) ;
#3724=ORIENTED_EDGE('',*,*,#2874,.T.) ;
#3725=ORIENTED_EDGE('',*,*,#2870,.F.) ;
#3726=ORIENTED_EDGE('',*,*,#2875,.T.) ;
#3727=ORIENTED_EDGE('',*,*,#2876,.T.) ;
#3728=ORIENTED_EDGE('',*,*,#2873,.F.) ;
#3729=ORIENTED_EDGE('',*,*,#2877,.T.) ;
#3730=ORIENTED_EDGE('',*,*,#2867,.F.) ;
#3731=ORIENTED_EDGE('',*,*,#2805,.T.) ;
#3732=ORIENTED_EDGE('',*,*,#2878,.T.) ;
#3733=ORIENTED_EDGE('',*,*,#2879,.T.) ;
#3734=ORIENTED_EDGE('',*,*,#2862,.F.) ;
#3735=ORIENTED_EDGE('',*,*,#2880,.T.) ;
#3736=ORIENTED_EDGE('',*,*,#2878,.F.) ;
#3737=ORIENTED_EDGE('',*,*,#2881,.T.) ;
#3738=ORIENTED_EDGE('',*,*,#2882,.T.) ;
#3739=ORIENTED_EDGE('',*,*,#2872,.F.) ;
#3740=ORIENTED_EDGE('',*,*,#2883,.T.) ;
#3741=ORIENTED_EDGE('',*,*,#2865,.F.) ;
#3742=ORIENTED_EDGE('',*,*,#2825,.T.) ;
#3743=ORIENTED_EDGE('',*,*,#2884,.T.) ;
#3744=ORIENTED_EDGE('',*,*,#2857,.F.) ;
#3745=ORIENTED_EDGE('',*,*,#2885,.T.) ;
#3746=ORIENTED_EDGE('',*,*,#2884,.F.) ;
#3747=ORIENTED_EDGE('',*,*,#2824,.T.) ;
#3748=ORIENTED_EDGE('',*,*,#2859,.F.) ;
#3749=ORIENTED_EDGE('',*,*,#2886,.T.) ;
#3750=ORIENTED_EDGE('',*,*,#2887,.T.) ;
#3751=ORIENTED_EDGE('',*,*,#2808,.T.) ;
#3752=ORIENTED_EDGE('',*,*,#2822,.T.) ;
#3753=ORIENTED_EDGE('',*,*,#2888,.T.) ;
#3754=ORIENTED_EDGE('',*,*,#2889,.T.) ;
#3755=ORIENTED_EDGE('',*,*,#2858,.F.) ;
#3756=ORIENTED_EDGE('',*,*,#2890,.T.) ;
#3757=ORIENTED_EDGE('',*,*,#2891,.T.) ;
#3758=ORIENTED_EDGE('',*,*,#2892,.T.) ;
#3759=ORIENTED_EDGE('',*,*,#2809,.T.) ;
#3760=ORIENTED_EDGE('',*,*,#2893,.T.) ;
#3761=ORIENTED_EDGE('',*,*,#2894,.T.) ;
#3762=ORIENTED_EDGE('',*,*,#2892,.F.) ;
#3763=ORIENTED_EDGE('',*,*,#2895,.T.) ;
#3764=ORIENTED_EDGE('',*,*,#2896,.T.) ;
#3765=ORIENTED_EDGE('',*,*,#2897,.T.) ;
#3766=ORIENTED_EDGE('',*,*,#2893,.F.) ;
#3767=ORIENTED_EDGE('',*,*,#2898,.T.) ;
#3768=ORIENTED_EDGE('',*,*,#2899,.T.) ;
#3769=ORIENTED_EDGE('',*,*,#2900,.T.) ;
#3770=ORIENTED_EDGE('',*,*,#2896,.F.) ;
#3771=ORIENTED_EDGE('',*,*,#2901,.T.) ;
#3772=ORIENTED_EDGE('',*,*,#2890,.F.) ;
#3773=ORIENTED_EDGE('',*,*,#2887,.F.) ;
#3774=ORIENTED_EDGE('',*,*,#2902,.T.) ;
#3775=ORIENTED_EDGE('',*,*,#2888,.F.) ;
#3776=ORIENTED_EDGE('',*,*,#2853,.F.) ;
#3777=ORIENTED_EDGE('',*,*,#2903,.T.) ;
#3778=ORIENTED_EDGE('',*,*,#2849,.F.) ;
#3779=ORIENTED_EDGE('',*,*,#2904,.F.) ;
#3780=ORIENTED_EDGE('',*,*,#2905,.T.) ;
#3781=ORIENTED_EDGE('',*,*,#2906,.F.) ;
#3782=ORIENTED_EDGE('',*,*,#2907,.F.) ;
#3783=ORIENTED_EDGE('',*,*,#2908,.F.) ;
#3784=ORIENTED_EDGE('',*,*,#2784,.F.) ;
#3785=ORIENTED_EDGE('',*,*,#2754,.T.) ;
#3786=ORIENTED_EDGE('',*,*,#2854,.F.) ;
#3787=ORIENTED_EDGE('',*,*,#2826,.T.) ;
#3788=ORIENTED_EDGE('',*,*,#2864,.F.) ;
#3789=ORIENTED_EDGE('',*,*,#2909,.F.) ;
#3790=ORIENTED_EDGE('',*,*,#2904,.T.) ;
#3791=ORIENTED_EDGE('',*,*,#2875,.F.) ;
#3792=ORIENTED_EDGE('',*,*,#2910,.F.) ;
#3793=ORIENTED_EDGE('',*,*,#2868,.F.) ;
#3794=ORIENTED_EDGE('',*,*,#2877,.F.) ;
#3795=ORIENTED_EDGE('',*,*,#2910,.T.) ;
#3796=ORIENTED_EDGE('',*,*,#2869,.F.) ;
#3797=ORIENTED_EDGE('',*,*,#2882,.F.) ;
#3798=ORIENTED_EDGE('',*,*,#2911,.T.) ;
#3799=ORIENTED_EDGE('',*,*,#2912,.T.) ;
#3800=ORIENTED_EDGE('',*,*,#2909,.T.) ;
#3801=ORIENTED_EDGE('',*,*,#2881,.F.) ;
#3802=ORIENTED_EDGE('',*,*,#2810,.T.) ;
#3803=ORIENTED_EDGE('',*,*,#2894,.F.) ;
#3804=ORIENTED_EDGE('',*,*,#2913,.T.) ;
#3805=ORIENTED_EDGE('',*,*,#2911,.F.) ;
#3806=ORIENTED_EDGE('',*,*,#2897,.F.) ;
#3807=ORIENTED_EDGE('',*,*,#2914,.F.) ;
#3808=ORIENTED_EDGE('',*,*,#2915,.F.) ;
#3809=ORIENTED_EDGE('',*,*,#2916,.F.) ;
#3810=ORIENTED_EDGE('',*,*,#2917,.F.) ;
#3811=ORIENTED_EDGE('',*,*,#2918,.F.) ;
#3812=ORIENTED_EDGE('',*,*,#2913,.F.) ;
#3813=ORIENTED_EDGE('',*,*,#2749,.T.) ;
#3814=ORIENTED_EDGE('',*,*,#2755,.T.) ;
#3815=ORIENTED_EDGE('',*,*,#2781,.T.) ;
#3816=ORIENTED_EDGE('',*,*,#2919,.F.) ;
#3817=ORIENTED_EDGE('',*,*,#2914,.T.) ;
#3818=ORIENTED_EDGE('',*,*,#2900,.F.) ;
#3819=ORIENTED_EDGE('',*,*,#2920,.T.) ;
#3820=ORIENTED_EDGE('',*,*,#2776,.T.) ;
#3821=ORIENTED_EDGE('',*,*,#2921,.T.) ;
#3822=ORIENTED_EDGE('',*,*,#2922,.T.) ;
#3823=ORIENTED_EDGE('',*,*,#2907,.T.) ;
#3824=ORIENTED_EDGE('',*,*,#2923,.T.) ;
#3825=ORIENTED_EDGE('',*,*,#2922,.F.) ;
#3826=ORIENTED_EDGE('',*,*,#2924,.T.) ;
#3827=ORIENTED_EDGE('',*,*,#2785,.F.) ;
#3828=ORIENTED_EDGE('',*,*,#2908,.T.) ;
#3829=ORIENTED_EDGE('',*,*,#2906,.T.) ;
#3830=ORIENTED_EDGE('',*,*,#2925,.T.) ;
#3831=ORIENTED_EDGE('',*,*,#2926,.T.) ;
#3832=ORIENTED_EDGE('',*,*,#2927,.T.) ;
#3833=ORIENTED_EDGE('',*,*,#2923,.F.) ;
#3834=ORIENTED_EDGE('',*,*,#2777,.T.) ;
#3835=ORIENTED_EDGE('',*,*,#2920,.F.) ;
#3836=ORIENTED_EDGE('',*,*,#2899,.F.) ;
#3837=ORIENTED_EDGE('',*,*,#2928,.T.) ;
#3838=ORIENTED_EDGE('',*,*,#2924,.F.) ;
#3839=ORIENTED_EDGE('',*,*,#2929,.F.) ;
#3840=ORIENTED_EDGE('',*,*,#2930,.F.) ;
#3841=ORIENTED_EDGE('',*,*,#2780,.T.) ;
#3842=ORIENTED_EDGE('',*,*,#2921,.F.) ;
#3843=ORIENTED_EDGE('',*,*,#2931,.F.) ;
#3844=ORIENTED_EDGE('',*,*,#2932,.F.) ;
#3845=ORIENTED_EDGE('',*,*,#2929,.T.) ;
#3846=ORIENTED_EDGE('',*,*,#2927,.F.) ;
#3847=ORIENTED_EDGE('',*,*,#2933,.F.) ;
#3848=ORIENTED_EDGE('',*,*,#2934,.F.) ;
#3849=ORIENTED_EDGE('',*,*,#2931,.T.) ;
#3850=ORIENTED_EDGE('',*,*,#2926,.F.) ;
#3851=ORIENTED_EDGE('',*,*,#2935,.F.) ;
#3852=ORIENTED_EDGE('',*,*,#2936,.F.) ;
#3853=ORIENTED_EDGE('',*,*,#2933,.T.) ;
#3854=ORIENTED_EDGE('',*,*,#2934,.T.) ;
#3855=ORIENTED_EDGE('',*,*,#2936,.T.) ;
#3856=ORIENTED_EDGE('',*,*,#2937,.T.) ;
#3857=ORIENTED_EDGE('',*,*,#2917,.T.) ;
#3858=ORIENTED_EDGE('',*,*,#2938,.T.) ;
#3859=ORIENTED_EDGE('',*,*,#2939,.T.) ;
#3860=ORIENTED_EDGE('',*,*,#2915,.T.) ;
#3861=ORIENTED_EDGE('',*,*,#2919,.T.) ;
#3862=ORIENTED_EDGE('',*,*,#2930,.T.) ;
#3863=ORIENTED_EDGE('',*,*,#2916,.T.) ;
#3864=ORIENTED_EDGE('',*,*,#2939,.F.) ;
#3865=ORIENTED_EDGE('',*,*,#2932,.T.) ;
#3866=ORIENTED_EDGE('',*,*,#2938,.F.) ;
#3867=ORIENTED_EDGE('',*,*,#2912,.F.) ;
#3868=ORIENTED_EDGE('',*,*,#2918,.T.) ;
#3869=ORIENTED_EDGE('',*,*,#2937,.F.) ;
#3870=ORIENTED_EDGE('',*,*,#2935,.T.) ;
#3871=ORIENTED_EDGE('',*,*,#2925,.F.) ;
#3872=ORIENTED_EDGE('',*,*,#2905,.F.) ;
#3873=ORIENTED_EDGE('',*,*,#2746,.T.) ;
#3874=ORIENTED_EDGE('',*,*,#2799,.F.) ;
#3875=ORIENTED_EDGE('',*,*,#2940,.F.) ;
#3876=ORIENTED_EDGE('',*,*,#2941,.T.) ;
#3877=ORIENTED_EDGE('',*,*,#2803,.T.) ;
#3878=ORIENTED_EDGE('',*,*,#2797,.F.) ;
#3879=ORIENTED_EDGE('',*,*,#2802,.F.) ;
#3880=ORIENTED_EDGE('',*,*,#2942,.T.) ;
#3881=ORIENTED_EDGE('',*,*,#2940,.T.) ;
#3882=ORIENTED_EDGE('',*,*,#2840,.F.) ;
#3883=ORIENTED_EDGE('',*,*,#2943,.F.) ;
#3884=ORIENTED_EDGE('',*,*,#2944,.T.) ;
#3885=ORIENTED_EDGE('',*,*,#2844,.T.) ;
#3886=ORIENTED_EDGE('',*,*,#2839,.F.) ;
#3887=ORIENTED_EDGE('',*,*,#2843,.F.) ;
#3888=ORIENTED_EDGE('',*,*,#2945,.T.) ;
#3889=ORIENTED_EDGE('',*,*,#2943,.T.) ;
#3890=ORIENTED_EDGE('',*,*,#2886,.F.) ;
#3891=ORIENTED_EDGE('',*,*,#2946,.F.) ;
#3892=ORIENTED_EDGE('',*,*,#2947,.F.) ;
#3893=ORIENTED_EDGE('',*,*,#2948,.T.) ;
#3894=ORIENTED_EDGE('',*,*,#2861,.F.) ;
#3895=ORIENTED_EDGE('',*,*,#2949,.F.) ;
#3896=ORIENTED_EDGE('',*,*,#2950,.T.) ;
#3897=ORIENTED_EDGE('',*,*,#2946,.T.) ;
#3898=ORIENTED_EDGE('',*,*,#2863,.F.) ;
#3899=ORIENTED_EDGE('',*,*,#2951,.F.) ;
#3900=ORIENTED_EDGE('',*,*,#2952,.F.) ;
#3901=ORIENTED_EDGE('',*,*,#2949,.T.) ;
#3902=ORIENTED_EDGE('',*,*,#2883,.F.) ;
#3903=ORIENTED_EDGE('',*,*,#2953,.F.) ;
#3904=ORIENTED_EDGE('',*,*,#2954,.T.) ;
#3905=ORIENTED_EDGE('',*,*,#2951,.T.) ;
#3906=ORIENTED_EDGE('',*,*,#2879,.F.) ;
#3907=ORIENTED_EDGE('',*,*,#2880,.F.) ;
#3908=ORIENTED_EDGE('',*,*,#2871,.F.) ;
#3909=ORIENTED_EDGE('',*,*,#2874,.F.) ;
#3910=ORIENTED_EDGE('',*,*,#2876,.F.) ;
#3911=ORIENTED_EDGE('',*,*,#2866,.F.) ;
#3912=ORIENTED_EDGE('',*,*,#2885,.F.) ;
#3913=ORIENTED_EDGE('',*,*,#2955,.F.) ;
#3914=ORIENTED_EDGE('',*,*,#2956,.F.) ;
#3915=ORIENTED_EDGE('',*,*,#2953,.T.) ;
#3916=ORIENTED_EDGE('',*,*,#2856,.F.) ;
#3917=ORIENTED_EDGE('',*,*,#2957,.F.) ;
#3918=ORIENTED_EDGE('',*,*,#2958,.T.) ;
#3919=ORIENTED_EDGE('',*,*,#2955,.T.) ;
#3920=ORIENTED_EDGE('',*,*,#2889,.F.) ;
#3921=ORIENTED_EDGE('',*,*,#2959,.F.) ;
#3922=ORIENTED_EDGE('',*,*,#2960,.F.) ;
#3923=ORIENTED_EDGE('',*,*,#2957,.T.) ;
#3924=ORIENTED_EDGE('',*,*,#2903,.F.) ;
#3925=ORIENTED_EDGE('',*,*,#2961,.F.) ;
#3926=ORIENTED_EDGE('',*,*,#2962,.T.) ;
#3927=ORIENTED_EDGE('',*,*,#2959,.T.) ;
#3928=ORIENTED_EDGE('',*,*,#2778,.T.) ;
#3929=ORIENTED_EDGE('',*,*,#2928,.F.) ;
#3930=ORIENTED_EDGE('',*,*,#2901,.F.) ;
#3931=ORIENTED_EDGE('',*,*,#2898,.F.) ;
#3932=ORIENTED_EDGE('',*,*,#2895,.F.) ;
#3933=ORIENTED_EDGE('',*,*,#2891,.F.) ;
#3934=ORIENTED_EDGE('',*,*,#2963,.F.) ;
#3935=ORIENTED_EDGE('',*,*,#2964,.F.) ;
#3936=ORIENTED_EDGE('',*,*,#2961,.T.) ;
#3937=ORIENTED_EDGE('',*,*,#2852,.F.) ;
#3938=ORIENTED_EDGE('',*,*,#2855,.F.) ;
#3939=ORIENTED_EDGE('',*,*,#2850,.F.) ;
#3940=ORIENTED_EDGE('',*,*,#2846,.F.) ;
#3941=ORIENTED_EDGE('',*,*,#2786,.F.) ;
#3942=ORIENTED_EDGE('',*,*,#2766,.T.) ;
#3943=ORIENTED_EDGE('',*,*,#2774,.T.) ;
#3944=ORIENTED_EDGE('',*,*,#2902,.F.) ;
#3945=ORIENTED_EDGE('',*,*,#2948,.F.) ;
#3946=ORIENTED_EDGE('',*,*,#2965,.T.) ;
#3947=ORIENTED_EDGE('',*,*,#2963,.T.) ;
#3948=ORIENTED_EDGE('',*,*,#2965,.F.) ;
#3949=ORIENTED_EDGE('',*,*,#2947,.T.) ;
#3950=ORIENTED_EDGE('',*,*,#2950,.F.) ;
#3951=ORIENTED_EDGE('',*,*,#2952,.T.) ;
#3952=ORIENTED_EDGE('',*,*,#2954,.F.) ;
#3953=ORIENTED_EDGE('',*,*,#2956,.T.) ;
#3954=ORIENTED_EDGE('',*,*,#2958,.F.) ;
#3955=ORIENTED_EDGE('',*,*,#2960,.T.) ;
#3956=ORIENTED_EDGE('',*,*,#2962,.F.) ;
#3957=ORIENTED_EDGE('',*,*,#2964,.T.) ;
#3958=ORIENTED_EDGE('',*,*,#2832,.F.) ;
#3959=ORIENTED_EDGE('',*,*,#2845,.F.) ;
#3960=ORIENTED_EDGE('',*,*,#2944,.F.) ;
#3961=ORIENTED_EDGE('',*,*,#2945,.F.) ;
#3962=ORIENTED_EDGE('',*,*,#2842,.F.) ;
#3963=ORIENTED_EDGE('',*,*,#2816,.F.) ;
#3964=ORIENTED_EDGE('',*,*,#2804,.F.) ;
#3965=ORIENTED_EDGE('',*,*,#2941,.F.) ;
#3966=ORIENTED_EDGE('',*,*,#2942,.F.) ;
#3967=ORIENTED_EDGE('',*,*,#2801,.F.) ;
#5092=CYLINDRICAL_SURFACE('',#5752,1.75) ;
#5093=CYLINDRICAL_SURFACE('',#5755,3.98) ;
#5094=CYLINDRICAL_SURFACE('',#5758,3.98) ;
#5095=CYLINDRICAL_SURFACE('',#5771,3.175) ;
#5096=CYLINDRICAL_SURFACE('',#5781,0.25) ;
#5097=CYLINDRICAL_SURFACE('',#5787,0.25) ;
#5098=CYLINDRICAL_SURFACE('',#5789,2.665) ;
#5099=CYLINDRICAL_SURFACE('',#5799,2.665) ;
#5100=CYLINDRICAL_SURFACE('',#5811,2.665) ;
#5101=CYLINDRICAL_SURFACE('',#5817,0.25) ;
#5102=CYLINDRICAL_SURFACE('',#5822,0.25) ;
#5103=CYLINDRICAL_SURFACE('',#5824,2.665) ;
#5104=CYLINDRICAL_SURFACE('',#5828,0.25) ;
#5105=CYLINDRICAL_SURFACE('',#5830,0.25) ;
#5106=CYLINDRICAL_SURFACE('',#5840,0.25) ;
#5107=CYLINDRICAL_SURFACE('',#5852,0.25) ;
#5108=CYLINDRICAL_SURFACE('',#5853,0.25) ;
#5109=CYLINDRICAL_SURFACE('',#5855,0.25) ;
#5110=CYLINDRICAL_SURFACE('',#5857,0.25) ;
#5111=CYLINDRICAL_SURFACE('',#5864,0.25) ;
#5112=CYLINDRICAL_SURFACE('',#5874,1.27) ;
#5113=CYLINDRICAL_SURFACE('',#5877,1.27) ;
#5114=CYLINDRICAL_SURFACE('',#5879,1.27) ;
#5115=CYLINDRICAL_SURFACE('',#5882,3.175) ;
#5116=CYLINDRICAL_SURFACE('',#5887,3.175) ;
#5117=CYLINDRICAL_SURFACE('',#5888,3.175) ;
#5118=CYLINDRICAL_SURFACE('',#5892,13.3598235398934) ;
#5119=CYLINDRICAL_SURFACE('',#5895,3.22733975942849) ;
#5120=CYLINDRICAL_SURFACE('',#5896,3.175) ;
#5121=CYLINDRICAL_SURFACE('',#5898,3.175) ;
#5122=CYLINDRICAL_SURFACE('',#5902,2.665) ;
#5123=CYLINDRICAL_SURFACE('',#5905,2.665) ;
#5124=CYLINDRICAL_SURFACE('',#5908,3.08595375255767) ;
#5125=CYLINDRICAL_SURFACE('',#5911,16.5858074534161) ;
#5126=CYLINDRICAL_SURFACE('',#5914,3.30499364382027) ;
#5127=CYLINDRICAL_SURFACE('',#5917,0.249999999999995) ;
#5128=CYLINDRICAL_SURFACE('',#5920,0.249999999999995) ;
#5233=ADVANCED_FACE('',(#508),#5092,.F.) ;
#5234=ADVANCED_FACE('',(#509),#5093,.F.) ;
#5235=ADVANCED_FACE('',(#510),#5094,.F.) ;
#5236=ADVANCED_FACE('',(#511),#396,.F.) ;
#5237=ADVANCED_FACE('',(#512,#337),#397,.F.) ;
#5238=ADVANCED_FACE('',(#513),#398,.F.) ;
#5239=ADVANCED_FACE('',(#514),#399,.F.) ;
#5240=ADVANCED_FACE('',(#515,#338),#400,.F.) ;
#5241=ADVANCED_FACE('',(#516),#401,.F.) ;
#5242=ADVANCED_FACE('',(#517,#339),#402,.T.) ;
#5243=ADVANCED_FACE('',(#518),#403,.T.) ;
#5244=ADVANCED_FACE('',(#519),#5095,.T.) ;
#5245=ADVANCED_FACE('',(#520),#404,.T.) ;
#5246=ADVANCED_FACE('',(#521),#176,.T.) ;
#5247=ADVANCED_FACE('',(#522),#5096,.T.) ;
#5248=ADVANCED_FACE('',(#523),#177,.T.) ;
#5249=ADVANCED_FACE('',(#524),#5097,.T.) ;
#5250=ADVANCED_FACE('',(#525),#405,.T.) ;
#5251=ADVANCED_FACE('',(#526),#5098,.F.) ;
#5252=ADVANCED_FACE('',(#527,#340,#341),#406,.T.) ;
#5253=ADVANCED_FACE('',(#528),#178,.T.) ;
#5254=ADVANCED_FACE('',(#529),#5099,.F.) ;
#5255=ADVANCED_FACE('',(#530),#179,.T.) ;
#5256=ADVANCED_FACE('',(#531,#342,#343),#407,.T.) ;
#5257=ADVANCED_FACE('',(#532),#5100,.F.) ;
#5258=ADVANCED_FACE('',(#533),#180,.T.) ;
#5259=ADVANCED_FACE('',(#534),#5101,.T.) ;
#5260=ADVANCED_FACE('',(#535),#181,.T.) ;
#5261=ADVANCED_FACE('',(#536),#5102,.T.) ;
#5262=ADVANCED_FACE('',(#537),#408,.T.) ;
#5263=ADVANCED_FACE('',(#538),#5103,.F.) ;
#5264=ADVANCED_FACE('',(#539),#170,.F.) ;
#5265=ADVANCED_FACE('',(#540),#5104,.T.) ;
#5266=ADVANCED_FACE('',(#541),#5105,.T.) ;
#5267=ADVANCED_FACE('',(#542),#182,.T.) ;
#5268=ADVANCED_FACE('',(#543),#183,.T.) ;
#5269=ADVANCED_FACE('',(#544),#184,.T.) ;
#5270=ADVANCED_FACE('',(#545),#5106,.T.) ;
#5271=ADVANCED_FACE('',(#546),#171,.F.) ;
#5272=ADVANCED_FACE('',(#547),#172,.F.) ;
#5273=ADVANCED_FACE('',(#548),#185,.T.) ;
#5274=ADVANCED_FACE('',(#549),#173,.F.) ;
#5275=ADVANCED_FACE('',(#550),#186,.T.) ;
#5276=ADVANCED_FACE('',(#551),#174,.F.) ;
#5277=ADVANCED_FACE('',(#552),#187,.T.) ;
#5278=ADVANCED_FACE('',(#553),#5107,.T.) ;
#5279=ADVANCED_FACE('',(#554),#5108,.T.) ;
#5280=ADVANCED_FACE('',(#555),#5109,.T.) ;
#5281=ADVANCED_FACE('',(#556),#5110,.T.) ;
#5282=ADVANCED_FACE('',(#557),#188,.T.) ;
#5283=ADVANCED_FACE('',(#558),#5111,.T.) ;
#5284=ADVANCED_FACE('',(#559),#175,.F.) ;
#5285=ADVANCED_FACE('',(#560),#168,.T.) ;
#5286=ADVANCED_FACE('',(#561),#169,.T.) ;
#5287=ADVANCED_FACE('',(#562,#344),#409,.T.) ;
#5288=ADVANCED_FACE('',(#563),#5112,.F.) ;
#5289=ADVANCED_FACE('',(#564),#410,.T.) ;
#5290=ADVANCED_FACE('',(#565),#5113,.F.) ;
#5291=ADVANCED_FACE('',(#566),#5114,.F.) ;
#5292=ADVANCED_FACE('',(#567,#345),#411,.F.) ;
#5293=ADVANCED_FACE('',(#568),#5115,.T.) ;
#5294=ADVANCED_FACE('',(#569),#189,.T.) ;
#5295=ADVANCED_FACE('',(#570),#5116,.T.) ;
#5296=ADVANCED_FACE('',(#571),#5117,.T.) ;
#5297=ADVANCED_FACE('',(#572),#412,.T.) ;
#5298=ADVANCED_FACE('',(#573),#413,.T.) ;
#5299=ADVANCED_FACE('',(#574),#5118,.T.) ;
#5300=ADVANCED_FACE('',(#575),#414,.T.) ;
#5301=ADVANCED_FACE('',(#576),#5119,.T.) ;
#5302=ADVANCED_FACE('',(#577),#5120,.T.) ;
#5303=ADVANCED_FACE('',(#578),#5121,.T.) ;
#5304=ADVANCED_FACE('',(#579),#190,.T.) ;
#5305=ADVANCED_FACE('',(#580,#346),#415,.T.) ;
#5306=ADVANCED_FACE('',(#581),#416,.T.) ;
#5307=ADVANCED_FACE('',(#582),#5122,.F.) ;
#5308=ADVANCED_FACE('',(#583),#417,.T.) ;
#5309=ADVANCED_FACE('',(#584),#5123,.F.) ;
#5310=ADVANCED_FACE('',(#585),#418,.T.) ;
#5311=ADVANCED_FACE('',(#586),#5124,.T.) ;
#5312=ADVANCED_FACE('',(#587),#419,.T.) ;
#5313=ADVANCED_FACE('',(#588),#5125,.T.) ;
#5314=ADVANCED_FACE('',(#589),#420,.T.) ;
#5315=ADVANCED_FACE('',(#590),#5126,.T.) ;
#5316=ADVANCED_FACE('',(#591),#421,.T.) ;
#5317=ADVANCED_FACE('',(#592),#5127,.T.) ;
#5318=ADVANCED_FACE('',(#593),#422,.T.) ;
#5319=ADVANCED_FACE('',(#594),#5128,.T.) ;
#5320=ADVANCED_FACE('',(#595,#347,#348,#349,#350),#423,.F.) ;
#5569=CLOSED_SHELL('',(#5233,#5234,#5235,#5236,#5237,#5238,#5239,#5240,
#5241,#5242,#5243,#5244,#5245,#5246,#5247,#5248,#5249,#5250,#5251,#5252,
#5253,#5254,#5255,#5256,#5257,#5258,#5259,#5260,#5261,#5262,#5263,#5264,
#5265,#5266,#5267,#5268,#5269,#5270,#5271,#5272,#5273,#5274,#5275,#5276,
#5277,#5278,#5279,#5280,#5281,#5282,#5283,#5284,#5285,#5286,#5287,#5288,
#5289,#5290,#5291,#5292,#5293,#5294,#5295,#5296,#5297,#5298,#5299,#5300,
#5301,#5302,#5303,#5304,#5305,#5306,#5307,#5308,#5309,#5310,#5311,#5312,
#5313,#5314,#5315,#5316,#5317,#5318,#5319,#5320)) ;
#5751=AXIS2_PLACEMENT_3D('',#8129,#6417,#6418) ;
#5752=AXIS2_PLACEMENT_3D('',#8130,#6419,#6420) ;
#5753=AXIS2_PLACEMENT_3D('',#8132,#6421,#6422) ;
#5754=AXIS2_PLACEMENT_3D('',#8135,#6424,#6425) ;
#5755=AXIS2_PLACEMENT_3D('',#8136,#6426,#6427) ;
#5756=AXIS2_PLACEMENT_3D('',#8138,#6428,#6429) ;
#5757=AXIS2_PLACEMENT_3D('',#8141,#6431,#6432) ;
#5758=AXIS2_PLACEMENT_3D('',#8142,#6433,#6434) ;
#5759=AXIS2_PLACEMENT_3D('',#8144,#6435,#6436) ;
#5760=AXIS2_PLACEMENT_3D('',#8147,#6438,#6439) ;
#5761=AXIS2_PLACEMENT_3D('',#8148,#6440,#6441) ;
#5762=AXIS2_PLACEMENT_3D('',#8151,#6442,#6443) ;
#5763=AXIS2_PLACEMENT_3D('',#8159,#6447,#6448) ;
#5764=AXIS2_PLACEMENT_3D('',#8161,#6450,#6451) ;
#5765=AXIS2_PLACEMENT_3D('',#8175,#6459,#6460) ;
#5766=AXIS2_PLACEMENT_3D('',#8179,#6463,#6464) ;
#5767=AXIS2_PLACEMENT_3D('',#8183,#6467,#6468) ;
#5768=AXIS2_PLACEMENT_3D('',#8187,#6471,#6472) ;
#5769=AXIS2_PLACEMENT_3D('',#8191,#6475,#6476) ;
#5770=AXIS2_PLACEMENT_3D('',#8197,#6480,#6481) ;
#5771=AXIS2_PLACEMENT_3D('',#8203,#6485,#6486) ;
#5772=AXIS2_PLACEMENT_3D('',#8205,#6487,#6488) ;
#5773=AXIS2_PLACEMENT_3D('',#8207,#6489,#6490) ;
#5774=AXIS2_PLACEMENT_3D('',#8210,#6492,#6493) ;
#5775=AXIS2_PLACEMENT_3D('',#8211,#6494,#6495) ;
#5776=AXIS2_PLACEMENT_3D('',#8234,#6497,#6498) ;
#5777=AXIS2_PLACEMENT_3D('',#8237,#6499,#6500) ;
#5778=AXIS2_PLACEMENT_3D('',#8239,#6501,#6502) ;
#5779=AXIS2_PLACEMENT_3D('',#8241,#6503,#6504) ;
#5780=AXIS2_PLACEMENT_3D('',#8242,#6505,#6506) ;
#5781=AXIS2_PLACEMENT_3D('',#8243,#6507,#6508) ;
#5782=AXIS2_PLACEMENT_3D('',#8246,#6509,#6510) ;
#5783=AXIS2_PLACEMENT_3D('',#8249,#6513,#6514) ;
#5784=AXIS2_PLACEMENT_3D('',#8252,#6515,#6516) ;
#5785=AXIS2_PLACEMENT_3D('',#8253,#6517,#6518) ;
#5786=AXIS2_PLACEMENT_3D('',#8254,#6519,#6520) ;
#5787=AXIS2_PLACEMENT_3D('',#8255,#6521,#6522) ;
#5788=AXIS2_PLACEMENT_3D('',#8258,#6525,#6526) ;
#5789=AXIS2_PLACEMENT_3D('',#8264,#6530,#6531) ;
#5790=AXIS2_PLACEMENT_3D('',#8267,#6533,#6534) ;
#5791=AXIS2_PLACEMENT_3D('',#8268,#6535,#6536) ;
#5792=AXIS2_PLACEMENT_3D('',#8271,#6537,#6538) ;
#5793=AXIS2_PLACEMENT_3D('',#8275,#6540,#6541) ;
#5794=AXIS2_PLACEMENT_3D('',#8282,#6545,#6546) ;
#5795=AXIS2_PLACEMENT_3D('',#8283,#6547,#6548) ;
#5796=AXIS2_PLACEMENT_3D('',#8285,#6549,#6550) ;
#5797=AXIS2_PLACEMENT_3D('',#8287,#6551,#6552) ;
#5798=AXIS2_PLACEMENT_3D('',#8288,#6553,#6554) ;
#5799=AXIS2_PLACEMENT_3D('',#8289,#6555,#6556) ;
#5800=AXIS2_PLACEMENT_3D('',#8292,#6558,#6559) ;
#5801=AXIS2_PLACEMENT_3D('',#8293,#6560,#6561) ;
#5802=AXIS2_PLACEMENT_3D('',#8295,#6562,#6563) ;
#5803=AXIS2_PLACEMENT_3D('',#8297,#6564,#6565) ;
#5804=AXIS2_PLACEMENT_3D('',#8299,#6566,#6567) ;
#5805=AXIS2_PLACEMENT_3D('',#8300,#6568,#6569) ;
#5806=AXIS2_PLACEMENT_3D('',#8301,#6570,#6571) ;
#5807=AXIS2_PLACEMENT_3D('',#8308,#6574,#6575) ;
#5808=AXIS2_PLACEMENT_3D('',#8312,#6577,#6578) ;
#5809=AXIS2_PLACEMENT_3D('',#8316,#6580,#6581) ;
#5810=AXIS2_PLACEMENT_3D('',#8320,#6583,#6584) ;
#5811=AXIS2_PLACEMENT_3D('',#8322,#6586,#6587) ;
#5812=AXIS2_PLACEMENT_3D('',#8325,#6589,#6590) ;
#5813=AXIS2_PLACEMENT_3D('',#8326,#6591,#6592) ;
#5814=AXIS2_PLACEMENT_3D('',#8328,#6593,#6594) ;
#5815=AXIS2_PLACEMENT_3D('',#8330,#6595,#6596) ;
#5816=AXIS2_PLACEMENT_3D('',#8331,#6597,#6598) ;
#5817=AXIS2_PLACEMENT_3D('',#8332,#6599,#6600) ;
#5818=AXIS2_PLACEMENT_3D('',#8334,#6601,#6602) ;
#5819=AXIS2_PLACEMENT_3D('',#8336,#6604,#6605) ;
#5820=AXIS2_PLACEMENT_3D('',#8338,#6606,#6607) ;
#5821=AXIS2_PLACEMENT_3D('',#8339,#6608,#6609) ;
#5822=AXIS2_PLACEMENT_3D('',#8340,#6610,#6611) ;
#5823=AXIS2_PLACEMENT_3D('',#8342,#6613,#6614) ;
#5824=AXIS2_PLACEMENT_3D('',#8348,#6618,#6619) ;
#5825=AXIS2_PLACEMENT_3D('',#8351,#6621,#6622) ;
#5826=AXIS2_PLACEMENT_3D('',#8378,#6623,#6624) ;
#5827=AXIS2_PLACEMENT_3D('',#8379,#6625,#6626) ;
#5828=AXIS2_PLACEMENT_3D('',#8380,#6627,#6628) ;
#5829=AXIS2_PLACEMENT_3D('',#8383,#6629,#6630) ;
#5830=AXIS2_PLACEMENT_3D('',#8386,#6633,#6634) ;
#5831=AXIS2_PLACEMENT_3D('',#8388,#6635,#6636) ;
#5832=AXIS2_PLACEMENT_3D('',#8391,#6638,#6639) ;
#5833=AXIS2_PLACEMENT_3D('',#8392,#6640,#6641) ;
#5834=AXIS2_PLACEMENT_3D('',#8393,#6642,#6643) ;
#5835=AXIS2_PLACEMENT_3D('',#8394,#6644,#6645) ;
#5836=AXIS2_PLACEMENT_3D('',#8395,#6646,#6647) ;
#5837=AXIS2_PLACEMENT_3D('',#8398,#6648,#6649) ;
#5838=AXIS2_PLACEMENT_3D('',#8439,#6650,#6651) ;
#5839=AXIS2_PLACEMENT_3D('',#8482,#6652,#6653) ;
#5840=AXIS2_PLACEMENT_3D('',#8483,#6654,#6655) ;
#5841=AXIS2_PLACEMENT_3D('',#8524,#6657,#6658) ;
#5842=AXIS2_PLACEMENT_3D('',#8593,#6659,#6660) ;
#5843=AXIS2_PLACEMENT_3D('',#8630,#6661,#6662) ;
#5844=AXIS2_PLACEMENT_3D('',#8633,#6663,#6664) ;
#5845=AXIS2_PLACEMENT_3D('',#8634,#6665,#6666) ;
#5846=AXIS2_PLACEMENT_3D('',#8635,#6667,#6668) ;
#5847=AXIS2_PLACEMENT_3D('',#8664,#6669,#6670) ;
#5848=AXIS2_PLACEMENT_3D('',#8666,#6671,#6672) ;
#5849=AXIS2_PLACEMENT_3D('',#8667,#6673,#6674) ;
#5850=AXIS2_PLACEMENT_3D('',#8701,#6675,#6676) ;
#5851=AXIS2_PLACEMENT_3D('',#8703,#6677,#6678) ;
#5852=AXIS2_PLACEMENT_3D('',#8716,#6679,#6680) ;
#5853=AXIS2_PLACEMENT_3D('',#8718,#6682,#6683) ;
#5854=AXIS2_PLACEMENT_3D('',#8721,#6685,#6686) ;
#5855=AXIS2_PLACEMENT_3D('',#8722,#6687,#6688) ;
#5856=AXIS2_PLACEMENT_3D('',#8724,#6689,#6690) ;
#5857=AXIS2_PLACEMENT_3D('',#8726,#6692,#6693) ;
#5858=AXIS2_PLACEMENT_3D('',#8728,#6694,#6695) ;
#5859=AXIS2_PLACEMENT_3D('',#8731,#6697,#6698) ;
#5860=AXIS2_PLACEMENT_3D('',#8732,#6699,#6700) ;
#5861=AXIS2_PLACEMENT_3D('',#8735,#6701,#6702) ;
#5862=AXIS2_PLACEMENT_3D('',#8736,#6703,#6704) ;
#5863=AXIS2_PLACEMENT_3D('',#8737,#6705,#6706) ;
#5864=AXIS2_PLACEMENT_3D('',#8738,#6707,#6708) ;
#5865=AXIS2_PLACEMENT_3D('',#8741,#6709,#6710) ;
#5866=AXIS2_PLACEMENT_3D('',#8791,#6713,#6714) ;
#5867=AXIS2_PLACEMENT_3D('',#8792,#6715,#6716) ;
#5868=AXIS2_PLACEMENT_3D('',#8793,#6717,#6718) ;
#5869=AXIS2_PLACEMENT_3D('',#8794,#6719,#6720) ;
#5870=AXIS2_PLACEMENT_3D('',#8795,#6721,#6722) ;
#5871=AXIS2_PLACEMENT_3D('',#8796,#6723,#6724) ;
#5872=AXIS2_PLACEMENT_3D('',#8797,#6725,#6726) ;
#5873=AXIS2_PLACEMENT_3D('',#8805,#6730,#6731) ;
#5874=AXIS2_PLACEMENT_3D('',#8807,#6733,#6734) ;
#5875=AXIS2_PLACEMENT_3D('',#8808,#6735,#6736) ;
#5876=AXIS2_PLACEMENT_3D('',#8809,#6737,#6738) ;
#5877=AXIS2_PLACEMENT_3D('',#8811,#6740,#6741) ;
#5878=AXIS2_PLACEMENT_3D('',#8813,#6742,#6743) ;
#5879=AXIS2_PLACEMENT_3D('',#8815,#6745,#6746) ;
#5880=AXIS2_PLACEMENT_3D('',#8817,#6748,#6749) ;
#5881=AXIS2_PLACEMENT_3D('',#8823,#6752,#6753) ;
#5882=AXIS2_PLACEMENT_3D('',#8827,#6756,#6757) ;
#5883=AXIS2_PLACEMENT_3D('',#8828,#6758,#6759) ;
#5884=AXIS2_PLACEMENT_3D('',#8829,#6760,#6761) ;
#5885=AXIS2_PLACEMENT_3D('',#8830,#6762,#6763) ;
#5886=AXIS2_PLACEMENT_3D('',#8833,#6764,#6765) ;
#5887=AXIS2_PLACEMENT_3D('',#8901,#6766,#6767) ;
#5888=AXIS2_PLACEMENT_3D('',#8903,#6769,#6770) ;
#5889=AXIS2_PLACEMENT_3D('',#8905,#6771,#6772) ;
#5890=AXIS2_PLACEMENT_3D('',#8930,#6774,#6775) ;
#5891=AXIS2_PLACEMENT_3D('',#8932,#6777,#6778) ;
#5892=AXIS2_PLACEMENT_3D('',#8936,#6781,#6782) ;
#5893=AXIS2_PLACEMENT_3D('',#8939,#6784,#6785) ;
#5894=AXIS2_PLACEMENT_3D('',#8940,#6786,#6787) ;
#5895=AXIS2_PLACEMENT_3D('',#8944,#6790,#6791) ;
#5896=AXIS2_PLACEMENT_3D('',#8969,#6793,#6794) ;
#5897=AXIS2_PLACEMENT_3D('',#8970,#6795,#6796) ;
#5898=AXIS2_PLACEMENT_3D('',#8989,#6797,#6798) ;
#5899=AXIS2_PLACEMENT_3D('',#9039,#6799,#6800) ;
#5900=AXIS2_PLACEMENT_3D('',#9040,#6801,#6802) ;
#5901=AXIS2_PLACEMENT_3D('',#9041,#6803,#6804) ;
#5902=AXIS2_PLACEMENT_3D('',#9045,#6807,#6808) ;
#5903=AXIS2_PLACEMENT_3D('',#9046,#6809,#6810) ;
#5904=AXIS2_PLACEMENT_3D('',#9047,#6811,#6812) ;
#5905=AXIS2_PLACEMENT_3D('',#9051,#6815,#6816) ;
#5906=AXIS2_PLACEMENT_3D('',#9052,#6817,#6818) ;
#5907=AXIS2_PLACEMENT_3D('',#9053,#6819,#6820) ;
#5908=AXIS2_PLACEMENT_3D('',#9059,#6824,#6825) ;
#5909=AXIS2_PLACEMENT_3D('',#9062,#6827,#6828) ;
#5910=AXIS2_PLACEMENT_3D('',#9063,#6829,#6830) ;
#5911=AXIS2_PLACEMENT_3D('',#9067,#6833,#6834) ;
#5912=AXIS2_PLACEMENT_3D('',#9070,#6836,#6837) ;
#5913=AXIS2_PLACEMENT_3D('',#9071,#6838,#6839) ;
#5914=AXIS2_PLACEMENT_3D('',#9075,#6842,#6843) ;
#5915=AXIS2_PLACEMENT_3D('',#9078,#6845,#6846) ;
#5916=AXIS2_PLACEMENT_3D('',#9079,#6847,#6848) ;
#5917=AXIS2_PLACEMENT_3D('',#9083,#6851,#6852) ;
#5918=AXIS2_PLACEMENT_3D('',#9086,#6854,#6855) ;
#5919=AXIS2_PLACEMENT_3D('',#9087,#6856,#6857) ;
#5920=AXIS2_PLACEMENT_3D('',#9091,#6860,#6861) ;
#5921=AXIS2_PLACEMENT_3D('',#9092,#6862,#6863) ;
#5922=AXIS2_PLACEMENT_3D('',#9093,#6864,#6865) ;
#6417=DIRECTION('axis',(0.,0.,1.)) ;
#6418=DIRECTION('refdir',(1.,0.,0.)) ;
#6419=DIRECTION('center_axis',(0.,0.,1.)) ;
#6420=DIRECTION('ref_axis',(1.,0.,0.)) ;
#6421=DIRECTION('center_axis',(0.,0.,1.)) ;
#6422=DIRECTION('ref_axis',(1.,0.,0.)) ;
#6423=DIRECTION('',(0.,0.,1.)) ;
#6424=DIRECTION('center_axis',(0.,0.,-1.)) ;
#6425=DIRECTION('ref_axis',(1.,0.,0.)) ;
#6426=DIRECTION('center_axis',(1.,0.,0.)) ;
#6427=DIRECTION('ref_axis',(0.,0.,-1.)) ;
#6428=DIRECTION('center_axis',(1.,0.,0.)) ;
#6429=DIRECTION('ref_axis',(0.,0.,-1.)) ;
#6430=DIRECTION('',(1.,0.,0.)) ;
#6431=DIRECTION('center_axis',(-1.,0.,0.)) ;
#6432=DIRECTION('ref_axis',(0.,0.,-1.)) ;
#6433=DIRECTION('center_axis',(1.,0.,0.)) ;
#6434=DIRECTION('ref_axis',(0.,0.,-1.)) ;
#6435=DIRECTION('center_axis',(1.,0.,0.)) ;
#6436=DIRECTION('ref_axis',(0.,0.,-1.)) ;
#6437=DIRECTION('',(1.,0.,0.)) ;
#6438=DIRECTION('center_axis',(-1.,0.,0.)) ;
#6439=DIRECTION('ref_axis',(0.,0.,-1.)) ;
#6440=DIRECTION('center_axis',(0.,1.,0.)) ;
#6441=DIRECTION('ref_axis',(0.,0.,1.)) ;
#6442=DIRECTION('center_axis',(0.,1.,0.)) ;
#6443=DIRECTION('ref_axis',(1.67369913353994E-16,0.,1.)) ;
#6444=DIRECTION('',(0.,0.,1.)) ;
#6445=DIRECTION('',(1.,0.,0.)) ;
#6446=DIRECTION('',(0.,0.,1.)) ;
#6447=DIRECTION('center_axis',(0.,1.,0.)) ;
#6448=DIRECTION('ref_axis',(-2.23159884471991E-16,-3.94494668997379E-17,
1.)) ;
#6449=DIRECTION('',(1.,0.,0.)) ;
#6450=DIRECTION('center_axis',(1.,0.,0.)) ;
#6451=DIRECTION('ref_axis',(0.,0.,-1.)) ;
#6452=DIRECTION('',(0.,-0.638189460570586,0.769879349259755)) ;
#6453=DIRECTION('',(0.,0.193633031896661,0.981074028276412)) ;
#6454=DIRECTION('',(0.,0.289220322623654,0.957262558017114)) ;
#6455=DIRECTION('',(0.,1.,0.)) ;
#6456=DIRECTION('',(0.,0.,-1.)) ;
#6457=DIRECTION('',(0.,-1.,0.)) ;
#6458=DIRECTION('',(0.,-0.989949493661166,0.141421356237312)) ;
#6459=DIRECTION('center_axis',(0.,0.981074028276412,-0.193633031896661)) ;
#6460=DIRECTION('ref_axis',(0.,0.193633031896661,0.981074028276412)) ;
#6461=DIRECTION('',(0.,0.193633031896661,0.981074028276412)) ;
#6462=DIRECTION('',(1.,0.,0.)) ;
#6463=DIRECTION('center_axis',(0.,0.957262558017114,-0.289220322623654)) ;
#6464=DIRECTION('ref_axis',(0.,0.289220322623654,0.957262558017114)) ;
#6465=DIRECTION('',(0.,0.289220322623654,0.957262558017114)) ;
#6466=DIRECTION('',(1.,0.,0.)) ;
#6467=DIRECTION('center_axis',(0.,0.,-1.)) ;
#6468=DIRECTION('ref_axis',(0.,1.,0.)) ;
#6469=DIRECTION('',(0.,1.,0.)) ;
#6470=DIRECTION('',(1.,0.,0.)) ;
#6471=DIRECTION('center_axis',(0.,-1.,0.)) ;
#6472=DIRECTION('ref_axis',(0.,0.,-1.)) ;
#6473=DIRECTION('',(-1.,0.,0.)) ;
#6474=DIRECTION('',(0.,0.,-1.)) ;
#6475=DIRECTION('center_axis',(1.,0.,0.)) ;
#6476=DIRECTION('ref_axis',(0.,0.,-1.)) ;
#6477=DIRECTION('',(0.,0.638189460570586,-0.769879349259755)) ;
#6478=DIRECTION('',(0.,0.989949493661166,-0.141421356237312)) ;
#6479=DIRECTION('',(0.,1.,0.)) ;
#6480=DIRECTION('center_axis',(0.,0.769879349259756,0.638189460570586)) ;
#6481=DIRECTION('ref_axis',(0.,-0.638189460570586,0.769879349259755)) ;
#6482=DIRECTION('',(0.,-0.638189460570586,0.769879349259755)) ;
#6483=DIRECTION('',(1.,0.,0.)) ;
#6484=DIRECTION('',(0.,0.638189460570586,-0.769879349259755)) ;
#6485=DIRECTION('center_axis',(0.,-0.638189460570586,0.769879349259756)) ;
#6486=DIRECTION('ref_axis',(0.707106781186548,0.54438690855706,0.451268095251245)) ;
#6487=DIRECTION('center_axis',(0.,-0.141421356237312,-0.989949493661166)) ;
#6488=DIRECTION('ref_axis',(0.,0.989949493661166,-0.141421356237312)) ;
#6489=DIRECTION('center_axis',(1.39759027204558E-15,-0.039937225530417,
0.999202190758674)) ;
#6490=DIRECTION('ref_axis',(0.,0.999202190758674,0.039937225530417)) ;
#6491=DIRECTION('',(0.,0.638189460570586,-0.769879349259755)) ;
#6492=DIRECTION('center_axis',(0.,-0.339205432400665,0.940712322992464)) ;
#6493=DIRECTION('ref_axis',(0.,0.940712322992464,0.339205432400665)) ;
#6494=DIRECTION('center_axis',(0.,0.141421356237312,0.989949493661166)) ;
#6495=DIRECTION('ref_axis',(0.,-0.989949493661166,0.141421356237312)) ;
#6496=DIRECTION('',(1.,0.,0.)) ;
#6497=DIRECTION('center_axis',(0.,-1.,0.)) ;
#6498=DIRECTION('ref_axis',(0.,0.,-1.)) ;
#6499=DIRECTION('center_axis',(-1.,0.,0.)) ;
#6500=DIRECTION('ref_axis',(0.,1.,0.)) ;
#6501=DIRECTION('center_axis',(0.,-1.,0.)) ;
#6502=DIRECTION('ref_axis',(-1.,0.,0.)) ;
#6503=DIRECTION('center_axis',(-1.,0.,0.)) ;
#6504=DIRECTION('ref_axis',(0.,0.,1.)) ;
#6505=DIRECTION('center_axis',(0.,1.,0.)) ;
#6506=DIRECTION('ref_axis',(-1.,0.,0.)) ;
#6507=DIRECTION('center_axis',(1.,0.,0.)) ;
#6508=DIRECTION('ref_axis',(0.,0.707106781186549,0.707106781186546)) ;
#6509=DIRECTION('center_axis',(-1.,0.,0.)) ;
#6510=DIRECTION('ref_axis',(0.,0.,1.)) ;
#6511=DIRECTION('',(-1.,0.,0.)) ;
#6512=DIRECTION('',(1.,0.,0.)) ;
#6513=DIRECTION('center_axis',(0.,-1.,0.)) ;
#6514=DIRECTION('ref_axis',(0.,0.,-1.)) ;
#6515=DIRECTION('center_axis',(1.,0.,0.)) ;
#6516=DIRECTION('ref_axis',(0.,0.,-1.)) ;
#6517=DIRECTION('center_axis',(0.,1.,0.)) ;
#6518=DIRECTION('ref_axis',(1.,0.,0.)) ;
#6519=DIRECTION('center_axis',(0.,-1.,0.)) ;
#6520=DIRECTION('ref_axis',(1.,0.,0.)) ;
#6521=DIRECTION('center_axis',(-1.,0.,0.)) ;
#6522=DIRECTION('ref_axis',(0.,0.707106781186549,-0.707106781186546)) ;
#6523=DIRECTION('',(1.,0.,0.)) ;
#6524=DIRECTION('',(-1.,0.,0.)) ;
#6525=DIRECTION('center_axis',(0.,0.,1.)) ;
#6526=DIRECTION('ref_axis',(1.,0.,0.)) ;
#6527=DIRECTION('',(0.,1.,0.)) ;
#6528=DIRECTION('',(1.,0.,0.)) ;
#6529=DIRECTION('',(0.,1.,0.)) ;
#6530=DIRECTION('center_axis',(0.,1.,0.)) ;
#6531=DIRECTION('ref_axis',(0.,0.,-1.)) ;
#6532=DIRECTION('',(0.,1.,0.)) ;
#6533=DIRECTION('center_axis',(0.,-1.,0.)) ;
#6534=DIRECTION('ref_axis',(0.,0.,-1.)) ;
#6535=DIRECTION('center_axis',(0.,1.,0.)) ;
#6536=DIRECTION('ref_axis',(1.,0.,0.)) ;
#6537=DIRECTION('center_axis',(0.,-1.,0.)) ;
#6538=DIRECTION('ref_axis',(-0.677879474603844,0.,-0.735173053036369)) ;
#6539=DIRECTION('',(0.707106781186548,0.,-0.707106781186547)) ;
#6540=DIRECTION('center_axis',(0.,-1.,0.)) ;
#6541=DIRECTION('ref_axis',(-0.921249561411385,0.,-0.388972037040364)) ;
#6542=DIRECTION('',(0.,0.,-1.)) ;
#6543=DIRECTION('',(-1.,0.,0.)) ;
#6544=DIRECTION('',(0.,0.,1.)) ;
#6545=DIRECTION('center_axis',(0.,1.,0.)) ;
#6546=DIRECTION('ref_axis',(1.,0.,0.)) ;
#6547=DIRECTION('center_axis',(0.,-1.,0.)) ;
#6548=DIRECTION('ref_axis',(0.,0.,-1.)) ;
#6549=DIRECTION('center_axis',(-1.,0.,0.)) ;
#6550=DIRECTION('ref_axis',(0.,0.,1.)) ;
#6551=DIRECTION('center_axis',(0.,-1.,0.)) ;
#6552=DIRECTION('ref_axis',(1.,0.,0.)) ;
#6553=DIRECTION('center_axis',(0.,-1.,0.)) ;
#6554=DIRECTION('ref_axis',(1.,0.,0.)) ;
#6555=DIRECTION('center_axis',(0.,1.,0.)) ;
#6556=DIRECTION('ref_axis',(1.,0.,0.)) ;
#6557=DIRECTION('',(0.,-1.,0.)) ;
#6558=DIRECTION('center_axis',(0.,-1.,0.)) ;
#6559=DIRECTION('ref_axis',(1.,0.,0.)) ;
#6560=DIRECTION('center_axis',(0.,-1.,0.)) ;
#6561=DIRECTION('ref_axis',(0.,0.,-1.)) ;
#6562=DIRECTION('center_axis',(0.,1.,0.)) ;
#6563=DIRECTION('ref_axis',(1.,0.,0.)) ;
#6564=DIRECTION('center_axis',(-1.,0.,0.)) ;
#6565=DIRECTION('ref_axis',(0.,0.,1.)) ;
#6566=DIRECTION('center_axis',(0.,-1.,0.)) ;
#6567=DIRECTION('ref_axis',(1.,0.,0.)) ;
#6568=DIRECTION('center_axis',(0.,-1.,0.)) ;
#6569=DIRECTION('ref_axis',(1.,0.,0.)) ;
#6570=DIRECTION('center_axis',(0.,1.,0.)) ;
#6571=DIRECTION('ref_axis',(1.,0.,0.)) ;
#6572=DIRECTION('',(-1.,0.,0.)) ;
#6573=DIRECTION('',(0.,0.,1.)) ;
#6574=DIRECTION('center_axis',(0.,-1.,0.)) ;
#6575=DIRECTION('ref_axis',(0.921249561411385,0.,-0.388972037040363)) ;
#6576=DIRECTION('',(0.707106781186548,0.,0.707106781186547)) ;
#6577=DIRECTION('center_axis',(0.,-1.,0.)) ;
#6578=DIRECTION('ref_axis',(0.677879474603844,0.,-0.735173053036369)) ;
#6579=DIRECTION('',(0.,0.,-1.)) ;
#6580=DIRECTION('center_axis',(0.,1.,0.)) ;
#6581=DIRECTION('ref_axis',(-1.,0.,0.)) ;
#6582=DIRECTION('',(-1.,0.,0.)) ;
#6583=DIRECTION('center_axis',(0.,1.,0.)) ;
#6584=DIRECTION('ref_axis',(1.,0.,0.)) ;
#6585=DIRECTION('',(1.,0.,0.)) ;
#6586=DIRECTION('center_axis',(0.,1.,0.)) ;
#6587=DIRECTION('ref_axis',(1.,0.,0.)) ;
#6588=DIRECTION('',(0.,-1.,0.)) ;
#6589=DIRECTION('center_axis',(0.,-1.,0.)) ;
#6590=DIRECTION('ref_axis',(1.,0.,0.)) ;
#6591=DIRECTION('center_axis',(0.,-1.,0.)) ;
#6592=DIRECTION('ref_axis',(0.,0.,-1.)) ;
#6593=DIRECTION('center_axis',(-1.,0.,0.)) ;
#6594=DIRECTION('ref_axis',(0.,1.,0.)) ;
#6595=DIRECTION('center_axis',(0.,-1.,0.)) ;
#6596=DIRECTION('ref_axis',(-1.,0.,0.)) ;
#6597=DIRECTION('center_axis',(-1.,0.,0.)) ;
#6598=DIRECTION('ref_axis',(0.,0.,1.)) ;
#6599=DIRECTION('center_axis',(1.,0.,0.)) ;
#6600=DIRECTION('ref_axis',(0.,0.707106781186549,0.707106781186546)) ;
#6601=DIRECTION('center_axis',(-1.,0.,0.)) ;
#6602=DIRECTION('ref_axis',(0.,0.,1.)) ;
#6603=DIRECTION('',(1.,0.,0.)) ;
#6604=DIRECTION('center_axis',(0.,-1.,0.)) ;
#6605=DIRECTION('ref_axis',(0.,0.,-1.)) ;
#6606=DIRECTION('center_axis',(1.,0.,0.)) ;
#6607=DIRECTION('ref_axis',(0.,0.,-1.)) ;
#6608=DIRECTION('center_axis',(0.,-1.,0.)) ;
#6609=DIRECTION('ref_axis',(1.,0.,0.)) ;
#6610=DIRECTION('center_axis',(-1.,0.,0.)) ;
#6611=DIRECTION('ref_axis',(0.,0.707106781186549,-0.707106781186546)) ;
#6612=DIRECTION('',(-1.,0.,0.)) ;
#6613=DIRECTION('center_axis',(0.,0.,1.)) ;
#6614=DIRECTION('ref_axis',(1.,0.,0.)) ;
#6615=DIRECTION('',(0.,1.,0.)) ;
#6616=DIRECTION('',(1.,0.,0.)) ;
#6617=DIRECTION('',(0.,1.,0.)) ;
#6618=DIRECTION('center_axis',(0.,1.,0.)) ;
#6619=DIRECTION('ref_axis',(0.,0.,-1.)) ;
#6620=DIRECTION('',(0.,1.,0.)) ;
#6621=DIRECTION('center_axis',(0.,-1.,0.)) ;
#6622=DIRECTION('ref_axis',(0.,0.,-1.)) ;
#6623=DIRECTION('center_axis',(0.,0.,-1.)) ;
#6624=DIRECTION('ref_axis',(0.,1.,0.)) ;
#6625=DIRECTION('center_axis',(0.,1.,0.)) ;
#6626=DIRECTION('ref_axis',(0.,0.,1.)) ;
#6627=DIRECTION('center_axis',(0.,-1.,0.)) ;
#6628=DIRECTION('ref_axis',(0.707106781186544,0.,0.707106781186551)) ;
#6629=DIRECTION('center_axis',(0.,1.,0.)) ;
#6630=DIRECTION('ref_axis',(0.,0.,1.)) ;
#6631=DIRECTION('',(0.,1.,0.)) ;
#6632=DIRECTION('',(0.,-1.,0.)) ;
#6633=DIRECTION('center_axis',(1.,0.,0.)) ;
#6634=DIRECTION('ref_axis',(0.,0.707106781186543,0.707106781186552)) ;
#6635=DIRECTION('center_axis',(1.,0.,0.)) ;
#6636=DIRECTION('ref_axis',(0.,1.,0.)) ;
#6637=DIRECTION('',(1.,0.,0.)) ;
#6638=DIRECTION('center_axis',(-1.,0.,0.)) ;
#6639=DIRECTION('ref_axis',(0.,0.,1.)) ;
#6640=DIRECTION('center_axis',(0.,0.,1.)) ;
#6641=DIRECTION('ref_axis',(1.,0.,0.)) ;
#6642=DIRECTION('center_axis',(0.,0.,-1.)) ;
#6643=DIRECTION('ref_axis',(-0.707106781186547,-0.707106781186548,0.)) ;
#6644=DIRECTION('center_axis',(0.,0.,1.)) ;
#6645=DIRECTION('ref_axis',(-0.707106781186547,-0.707106781186548,0.)) ;
#6646=DIRECTION('center_axis',(0.,1.,0.)) ;
#6647=DIRECTION('ref_axis',(0.,0.,1.)) ;
#6648=DIRECTION('center_axis',(0.,1.,0.)) ;
#6649=DIRECTION('ref_axis',(0.921249561411386,0.,-0.388972037040363)) ;
#6650=DIRECTION('center_axis',(0.,1.,0.)) ;
#6651=DIRECTION('ref_axis',(0.,0.,1.)) ;
#6652=DIRECTION('center_axis',(0.,1.,0.)) ;
#6653=DIRECTION('ref_axis',(-0.921249561411385,0.,-0.388972037040364)) ;
#6654=DIRECTION('center_axis',(-0.707106781186548,0.,0.707106781186547)) ;
#6655=DIRECTION('ref_axis',(-0.499999999999999,0.707106781186549,-0.499999999999999)) ;
#6656=DIRECTION('',(-0.707106781186548,0.,0.707106781186547)) ;
#6657=DIRECTION('center_axis',(-0.751890603952275,6.67813008405704E-15,
-0.659287888322153)) ;
#6658=DIRECTION('ref_axis',(8.88178419700124E-15,1.,0.)) ;
#6659=DIRECTION('center_axis',(-0.791256109639887,-1.01273265766357E-13,
0.611484888576612)) ;
#6660=DIRECTION('ref_axis',(-4.44089209850062E-15,1.,1.59872115546022E-13)) ;
#6661=DIRECTION('center_axis',(0.,1.,0.)) ;
#6662=DIRECTION('ref_axis',(2.78699993901511E-15,0.,-1.)) ;
#6663=DIRECTION('center_axis',(-0.79125610963988,0.,-0.61148488857662)) ;
#6664=DIRECTION('ref_axis',(0.,1.,0.)) ;
#6665=DIRECTION('center_axis',(0.,1.,0.)) ;
#6666=DIRECTION('ref_axis',(6.69381353752835E-17,0.,-1.)) ;
#6667=DIRECTION('center_axis',(0.,-1.,0.)) ;
#6668=DIRECTION('ref_axis',(6.69381353752835E-17,0.,-1.)) ;
#6669=DIRECTION('center_axis',(0.,1.,0.)) ;
#6670=DIRECTION('ref_axis',(0.,0.,1.)) ;
#6671=DIRECTION('center_axis',(-0.751890603952276,-5.03317541149096E-15,
0.659287888322151)) ;
#6672=DIRECTION('ref_axis',(8.88178419700124E-15,1.,1.77635683940025E-14)) ;
#6673=DIRECTION('center_axis',(0.,1.,0.)) ;
#6674=DIRECTION('ref_axis',(-0.677879474603844,0.,-0.735173053036369)) ;
#6675=DIRECTION('center_axis',(0.,1.,0.)) ;
#6676=DIRECTION('ref_axis',(0.,0.,1.)) ;
#6677=DIRECTION('center_axis',(0.,1.,0.)) ;
#6678=DIRECTION('ref_axis',(0.677879474603844,0.,-0.735173053036369)) ;
#6679=DIRECTION('center_axis',(-0.707106781186548,0.,-0.707106781186547)) ;
#6680=DIRECTION('ref_axis',(0.499999999999999,0.707106781186549,-0.499999999999999)) ;
#6681=DIRECTION('',(-0.707106781186548,0.,-0.707106781186547)) ;
#6682=DIRECTION('center_axis',(0.,0.,1.)) ;
#6683=DIRECTION('ref_axis',(-0.707106781186552,0.707106781186543,0.)) ;
#6684=DIRECTION('',(0.,0.,1.)) ;
#6685=DIRECTION('center_axis',(0.,0.,-1.)) ;
#6686=DIRECTION('ref_axis',(-1.,0.,0.)) ;
#6687=DIRECTION('center_axis',(0.,0.,-1.)) ;
#6688=DIRECTION('ref_axis',(0.707106781186552,0.707106781186543,0.)) ;
#6689=DIRECTION('center_axis',(0.,0.,-1.)) ;
#6690=DIRECTION('ref_axis',(0.,1.,0.)) ;
#6691=DIRECTION('',(0.,0.,-1.)) ;
#6692=DIRECTION('center_axis',(1.,0.,0.)) ;
#6693=DIRECTION('ref_axis',(0.,0.707106781186543,0.707106781186552)) ;
#6694=DIRECTION('center_axis',(1.,0.,0.)) ;
#6695=DIRECTION('ref_axis',(0.,1.,0.)) ;
#6696=DIRECTION('',(1.,0.,0.)) ;
#6697=DIRECTION('center_axis',(-1.,0.,0.)) ;
#6698=DIRECTION('ref_axis',(0.,0.,1.)) ;
#6699=DIRECTION('center_axis',(0.,0.,1.)) ;
#6700=DIRECTION('ref_axis',(1.,0.,0.)) ;
#6701=DIRECTION('center_axis',(0.,-1.,0.)) ;
#6702=DIRECTION('ref_axis',(0.,0.,1.)) ;
#6703=DIRECTION('center_axis',(0.,0.,-1.)) ;
#6704=DIRECTION('ref_axis',(0.707106781186547,-0.707106781186548,0.)) ;
#6705=DIRECTION('center_axis',(0.,0.,1.)) ;
#6706=DIRECTION('ref_axis',(0.707106781186547,-0.707106781186548,0.)) ;
#6707=DIRECTION('center_axis',(0.,-1.,0.)) ;
#6708=DIRECTION('ref_axis',(-0.707106781186541,0.,0.707106781186554)) ;
#6709=DIRECTION('center_axis',(0.,-1.,0.)) ;
#6710=DIRECTION('ref_axis',(0.,0.,1.)) ;
#6711=DIRECTION('',(0.,-1.,0.)) ;
#6712=DIRECTION('',(0.,1.,0.)) ;
#6713=DIRECTION('center_axis',(0.,-0.039937225530417,0.999202190758674)) ;
#6714=DIRECTION('ref_axis',(0.,0.999202190758674,0.039937225530417)) ;
#6715=DIRECTION('center_axis',(0.,0.,-1.)) ;
#6716=DIRECTION('ref_axis',(1.46109022176344E-16,1.,0.)) ;
#6717=DIRECTION('center_axis',(-0.816496580927738,-0.408248290463869,-0.408248290463833)) ;
#6718=DIRECTION('ref_axis',(-0.577350269189608,0.577350269189647,0.577350269189622)) ;
#6719=DIRECTION('center_axis',(0.,1.,0.)) ;
#6720=DIRECTION('ref_axis',(-1.,0.,-1.77635683940029E-14)) ;
#6721=DIRECTION('center_axis',(-0.816496580927738,0.408248290463869,0.408248290463833)) ;
#6722=DIRECTION('ref_axis',(0.577350269189608,0.577350269189647,0.577350269189622)) ;
#6723=DIRECTION('center_axis',(0.,1.,0.)) ;
#6724=DIRECTION('ref_axis',(-1.77635683940029E-14,0.,1.)) ;
#6725=DIRECTION('center_axis',(1.,0.,0.)) ;
#6726=DIRECTION('ref_axis',(0.,0.,-1.)) ;
#6727=DIRECTION('',(0.,0.,1.)) ;
#6728=DIRECTION('',(0.,1.,0.)) ;
#6729=DIRECTION('',(0.,-0.287347885566346,-0.957826285221151)) ;
#6730=DIRECTION('center_axis',(-1.,0.,0.)) ;
#6731=DIRECTION('ref_axis',(0.,0.988836773758751,-0.14900280152529)) ;
#6732=DIRECTION('',(0.,0.,-1.)) ;
#6733=DIRECTION('center_axis',(0.,0.,1.)) ;
#6734=DIRECTION('ref_axis',(-0.707106781186547,-0.707106781186548,0.)) ;
#6735=DIRECTION('center_axis',(0.707106781186548,0.,0.707106781186547)) ;
#6736=DIRECTION('ref_axis',(-0.707106781186547,0.,0.707106781186548)) ;
#6737=DIRECTION('center_axis',(0.,1.,0.)) ;
#6738=DIRECTION('ref_axis',(1.,0.,0.)) ;
#6739=DIRECTION('',(-1.,0.,0.)) ;
#6740=DIRECTION('center_axis',(1.,0.,0.)) ;
#6741=DIRECTION('ref_axis',(0.,-0.707106781186546,0.707106781186549)) ;
#6742=DIRECTION('center_axis',(-0.707106781186548,0.,0.707106781186547)) ;
#6743=DIRECTION('ref_axis',(-0.707106781186547,0.,-0.707106781186548)) ;
#6744=DIRECTION('',(1.,0.,0.)) ;
#6745=DIRECTION('center_axis',(0.,0.,-1.)) ;
#6746=DIRECTION('ref_axis',(0.707106781186547,-0.707106781186548,0.)) ;
#6747=DIRECTION('',(0.,0.,-1.)) ;
#6748=DIRECTION('center_axis',(1.,0.,0.)) ;
#6749=DIRECTION('ref_axis',(0.,0.,-1.)) ;
#6750=DIRECTION('',(0.,-0.638189460570586,0.769879349259755)) ;
#6751=DIRECTION('',(0.,0.,1.)) ;
#6752=DIRECTION('center_axis',(1.,0.,0.)) ;
#6753=DIRECTION('ref_axis',(0.,0.988836773758751,-0.14900280152529)) ;
#6754=DIRECTION('',(0.,0.287347885566346,0.957826285221151)) ;
#6755=DIRECTION('',(0.,1.,0.)) ;
#6756=DIRECTION('center_axis',(0.,-0.638189460570586,0.769879349259756)) ;
#6757=DIRECTION('ref_axis',(-0.707106781186548,0.544386908557059,0.451268095251246)) ;
#6758=DIRECTION('center_axis',(0.,0.339205432400664,-0.940712322992464)) ;
#6759=DIRECTION('ref_axis',(0.,-0.940712322992464,-0.339205432400664)) ;
#6760=DIRECTION('center_axis',(0.,-0.141421356237312,-0.989949493661166)) ;
#6761=DIRECTION('ref_axis',(0.,0.989949493661166,-0.141421356237312)) ;
#6762=DIRECTION('center_axis',(1.,0.,0.)) ;
#6763=DIRECTION('ref_axis',(0.,0.,-1.)) ;
#6764=DIRECTION('center_axis',(1.,0.,0.)) ;
#6765=DIRECTION('ref_axis',(0.,0.988836773758751,-0.14900280152529)) ;
#6766=DIRECTION('center_axis',(0.,0.,1.)) ;
#6767=DIRECTION('ref_axis',(0.707106781186548,0.707106781186548,0.)) ;
#6768=DIRECTION('',(0.,0.,1.)) ;
#6769=DIRECTION('center_axis',(0.,0.287347885566346,0.957826285221151)) ;
#6770=DIRECTION('ref_axis',(0.707106781186548,0.677285461478596,-0.203185638443579)) ;
#6771=DIRECTION('center_axis',(0.,0.,1.)) ;
#6772=DIRECTION('ref_axis',(-1.33971753756687E-15,1.,0.)) ;
#6773=DIRECTION('',(0.,0.287347885566346,0.957826285221151)) ;
#6774=DIRECTION('center_axis',(0.,0.141421356237312,0.989949493661166)) ;
#6775=DIRECTION('ref_axis',(0.,-0.989949493661166,0.141421356237312)) ;
#6776=DIRECTION('',(1.,0.,0.)) ;
#6777=DIRECTION('center_axis',(0.,1.,0.)) ;
#6778=DIRECTION('ref_axis',(0.,0.,1.)) ;
#6779=DIRECTION('',(1.,0.,0.)) ;
#6780=DIRECTION('',(0.,0.,-1.)) ;
#6781=DIRECTION('center_axis',(1.,0.,0.)) ;
#6782=DIRECTION('ref_axis',(0.,0.958771613297587,-0.284177749893868)) ;
#6783=DIRECTION('',(1.,0.,0.)) ;
#6784=DIRECTION('center_axis',(-1.,0.,0.)) ;
#6785=DIRECTION('ref_axis',(0.,0.988836773758751,-0.14900280152529)) ;
#6786=DIRECTION('center_axis',(0.,0.957826285221151,-0.287347885566346)) ;
#6787=DIRECTION('ref_axis',(0.,0.287347885566346,0.957826285221151)) ;
#6788=DIRECTION('',(1.,0.,0.)) ;
#6789=DIRECTION('',(0.,-0.287347885566346,-0.957826285221151)) ;
#6790=DIRECTION('center_axis',(1.,0.,0.)) ;
#6791=DIRECTION('ref_axis',(0.,0.00800353445718605,-0.999967971205174)) ;
#6792=DIRECTION('',(1.,0.,0.)) ;
#6793=DIRECTION('center_axis',(0.,0.287347885566346,0.957826285221151)) ;
#6794=DIRECTION('ref_axis',(-0.707106781186548,0.677285461478596,-0.203185638443579)) ;
#6795=DIRECTION('center_axis',(0.,0.,1.)) ;
#6796=DIRECTION('ref_axis',(1.33971753756687E-15,1.,0.)) ;
#6797=DIRECTION('center_axis',(0.,0.,1.)) ;
#6798=DIRECTION('ref_axis',(-0.707106781186548,0.707106781186548,0.)) ;
#6799=DIRECTION('center_axis',(1.,0.,0.)) ;
#6800=DIRECTION('ref_axis',(0.,0.,-1.)) ;
#6801=DIRECTION('center_axis',(0.,0.,-1.)) ;
#6802=DIRECTION('ref_axis',(0.,1.,0.)) ;
#6803=DIRECTION('center_axis',(0.,0.,-1.)) ;
#6804=DIRECTION('ref_axis',(-1.,0.,0.)) ;
#6805=DIRECTION('',(0.,1.,0.)) ;
#6806=DIRECTION('',(-1.,0.,0.)) ;
#6807=DIRECTION('center_axis',(0.,1.,0.)) ;
#6808=DIRECTION('ref_axis',(0.,0.,1.)) ;
#6809=DIRECTION('center_axis',(0.,-1.,0.)) ;
#6810=DIRECTION('ref_axis',(0.,0.,1.)) ;
#6811=DIRECTION('center_axis',(0.,0.,-1.)) ;
#6812=DIRECTION('ref_axis',(-1.,0.,0.)) ;
#6813=DIRECTION('',(0.,1.,0.)) ;
#6814=DIRECTION('',(-1.,0.,0.)) ;
#6815=DIRECTION('center_axis',(0.,1.,0.)) ;
#6816=DIRECTION('ref_axis',(0.,0.,1.)) ;
#6817=DIRECTION('center_axis',(0.,-1.,0.)) ;
#6818=DIRECTION('ref_axis',(0.,0.,1.)) ;
#6819=DIRECTION('center_axis',(-1.,0.,0.)) ;
#6820=DIRECTION('ref_axis',(0.,0.,1.)) ;
#6821=DIRECTION('',(0.,1.,0.)) ;
#6822=DIRECTION('',(0.,0.,-1.)) ;
#6823=DIRECTION('',(0.,1.,0.)) ;
#6824=DIRECTION('center_axis',(0.,1.,0.)) ;
#6825=DIRECTION('ref_axis',(-0.692126626006242,0.,-0.721776096565421)) ;
#6826=DIRECTION('',(0.,1.,0.)) ;
#6827=DIRECTION('center_axis',(0.,1.,0.)) ;
#6828=DIRECTION('ref_axis',(-0.692126626006242,0.,-0.721776096565421)) ;
#6829=DIRECTION('center_axis',(-0.707106781186547,0.,-0.707106781186548)) ;
#6830=DIRECTION('ref_axis',(-0.707106781186548,0.,0.707106781186547)) ;
#6831=DIRECTION('',(0.,1.,0.)) ;
#6832=DIRECTION('',(0.707106781186548,0.,-0.707106781186547)) ;
#6833=DIRECTION('center_axis',(0.,1.,0.)) ;
#6834=DIRECTION('ref_axis',(0.705422393987226,0.,-0.708787165559119)) ;
#6835=DIRECTION('',(0.,1.,0.)) ;
#6836=DIRECTION('center_axis',(0.,1.,0.)) ;
#6837=DIRECTION('ref_axis',(0.705422393987226,0.,-0.708787165559119)) ;
#6838=DIRECTION('center_axis',(0.707106781186547,0.,-0.707106781186548)) ;
#6839=DIRECTION('ref_axis',(-0.707106781186548,0.,-0.707106781186547)) ;
#6840=DIRECTION('',(0.,1.,0.)) ;
#6841=DIRECTION('',(0.707106781186548,0.,0.707106781186547)) ;
#6842=DIRECTION('center_axis',(0.,1.,0.)) ;
#6843=DIRECTION('ref_axis',(0.999778380675594,0.,-0.0210520672069664)) ;
#6844=DIRECTION('',(0.,1.,0.)) ;
#6845=DIRECTION('center_axis',(0.,1.,0.)) ;
#6846=DIRECTION('ref_axis',(0.999778380675594,0.,-0.0210520672069664)) ;
#6847=DIRECTION('center_axis',(1.,0.,0.)) ;
#6848=DIRECTION('ref_axis',(0.,0.,-1.)) ;
#6849=DIRECTION('',(0.,1.,0.)) ;
#6850=DIRECTION('',(0.,0.,1.)) ;
#6851=DIRECTION('center_axis',(0.,1.,0.)) ;
#6852=DIRECTION('ref_axis',(-1.77635683940029E-14,0.,1.)) ;
#6853=DIRECTION('',(0.,1.,0.)) ;
#6854=DIRECTION('center_axis',(0.,1.,0.)) ;
#6855=DIRECTION('ref_axis',(-1.77635683940029E-14,0.,1.)) ;
#6856=DIRECTION('center_axis',(0.,0.,1.)) ;
#6857=DIRECTION('ref_axis',(1.,0.,0.)) ;
#6858=DIRECTION('',(0.,1.,0.)) ;
#6859=DIRECTION('',(-1.,0.,0.)) ;
#6860=DIRECTION('center_axis',(0.,1.,0.)) ;
#6861=DIRECTION('ref_axis',(-1.,0.,-1.77635683940029E-14)) ;
#6862=DIRECTION('center_axis',(0.,1.,0.)) ;
#6863=DIRECTION('ref_axis',(-1.,0.,-1.77635683940029E-14)) ;
#6864=DIRECTION('center_axis',(0.,1.,0.)) ;
#6865=DIRECTION('ref_axis',(1.,0.,0.)) ;
#8129=CARTESIAN_POINT('',(0.,0.,0.)) ;
#8130=CARTESIAN_POINT('Origin',(0.475,7.535,-29.)) ;
#8131=CARTESIAN_POINT('',(-1.275,7.535,-28.55)) ;
#8132=CARTESIAN_POINT('Origin',(0.475,7.535,-28.55)) ;
#8133=CARTESIAN_POINT('',(-1.275,7.535,-20.)) ;
#8134=CARTESIAN_POINT('',(-1.275,7.535,-29.)) ;
#8135=CARTESIAN_POINT('Origin',(0.475,7.535,-20.)) ;
#8136=CARTESIAN_POINT('Origin',(-30.,17.565,27.14)) ;
#8137=CARTESIAN_POINT('',(-9.5,17.565,31.12)) ;
#8138=CARTESIAN_POINT('Origin',(-9.5,17.565,27.14)) ;
#8139=CARTESIAN_POINT('',(-6.35,17.565,31.12)) ;
#8140=CARTESIAN_POINT('',(-30.,17.565,31.12)) ;
#8141=CARTESIAN_POINT('Origin',(-6.35,17.565,27.14)) ;
#8142=CARTESIAN_POINT('Origin',(-30.,17.565,27.14)) ;
#8143=CARTESIAN_POINT('',(6.35,17.565,31.12)) ;
#8144=CARTESIAN_POINT('Origin',(6.35,17.565,27.14)) ;
#8145=CARTESIAN_POINT('',(9.5,17.565,31.12)) ;
#8146=CARTESIAN_POINT('',(-30.,17.565,31.12)) ;
#8147=CARTESIAN_POINT('Origin',(9.5,17.565,27.14)) ;
#8148=CARTESIAN_POINT('Origin',(-6.35,28.75,26.)) ;
#8149=CARTESIAN_POINT('',(-6.35,28.75,33.2188933909875)) ;
#8150=CARTESIAN_POINT('',(-6.325,28.75,33.2190476190476)) ;
#8151=CARTESIAN_POINT('Origin',(-6.325,28.75,28.2440359709998)) ;
#8152=CARTESIAN_POINT('',(-6.35,28.75,26.)) ;
#8153=CARTESIAN_POINT('',(-6.35,28.75,26.)) ;
#8154=CARTESIAN_POINT('',(6.35,28.75,26.)) ;
#8155=CARTESIAN_POINT('',(-6.35,28.75,26.)) ;
#8156=CARTESIAN_POINT('',(6.35,28.75,33.2188933909875)) ;
#8157=CARTESIAN_POINT('',(6.35,28.75,26.)) ;
#8158=CARTESIAN_POINT('',(6.325,28.75,33.2190476190476)) ;
#8159=CARTESIAN_POINT('Origin',(6.325,28.75,28.2440359709998)) ;
#8160=CARTESIAN_POINT('',(-7.925,28.75,33.2190476190476)) ;
#8161=CARTESIAN_POINT('Origin',(6.35,14.875,7.)) ;
#8162=CARTESIAN_POINT('',(6.35,28.5998549795853,33.4000207172021)) ;
#8163=CARTESIAN_POINT('',(6.35,35.4862056496714,25.0926770517013)) ;
#8164=CARTESIAN_POINT('',(6.35,28.,22.2)) ;
#8165=CARTESIAN_POINT('',(6.35,28.,22.2)) ;
#8166=CARTESIAN_POINT('',(6.35,15.25,-20.)) ;
#8167=CARTESIAN_POINT('',(6.35,15.25,-20.)) ;
#8168=CARTESIAN_POINT('',(6.35,1.,-20.)) ;
#8169=CARTESIAN_POINT('',(6.35,1.,-20.)) ;
#8170=CARTESIAN_POINT('',(6.35,1.,33.5)) ;
#8171=CARTESIAN_POINT('',(6.35,1.,34.)) ;
#8172=CARTESIAN_POINT('',(6.35,27.9,33.5)) ;
#8173=CARTESIAN_POINT('',(6.35,7.4375,33.5)) ;
#8174=CARTESIAN_POINT('',(6.35,23.72275,34.09675)) ;
#8175=CARTESIAN_POINT('Origin',(-6.35,28.,22.2)) ;
#8176=CARTESIAN_POINT('',(-6.35,28.,22.2)) ;
#8177=CARTESIAN_POINT('',(-6.35,28.,22.2)) ;
#8178=CARTESIAN_POINT('',(-6.35,28.,22.2)) ;
#8179=CARTESIAN_POINT('Origin',(-6.35,15.25,-20.)) ;
#8180=CARTESIAN_POINT('',(-6.35,15.25,-20.)) ;
#8181=CARTESIAN_POINT('',(-6.35,15.25,-20.)) ;
#8182=CARTESIAN_POINT('',(-6.35,15.25,-20.)) ;
#8183=CARTESIAN_POINT('Origin',(-6.35,1.,-20.)) ;
#8184=CARTESIAN_POINT('',(-6.35,1.,-20.)) ;
#8185=CARTESIAN_POINT('',(-6.35,1.,-20.)) ;
#8186=CARTESIAN_POINT('',(-6.35,1.,-20.)) ;
#8187=CARTESIAN_POINT('Origin',(-6.35,1.,34.)) ;
#8188=CARTESIAN_POINT('',(-6.35,1.,33.5)) ;
#8189=CARTESIAN_POINT('',(-15.425,1.,33.5)) ;
#8190=CARTESIAN_POINT('',(-6.35,1.,34.)) ;
#8191=CARTESIAN_POINT('Origin',(-6.35,14.875,7.)) ;
#8192=CARTESIAN_POINT('',(-6.35,28.5998549795853,33.4000207172021)) ;
#8193=CARTESIAN_POINT('',(-6.35,35.4862056496714,25.0926770517013)) ;
#8194=CARTESIAN_POINT('',(-6.35,27.9,33.5)) ;
#8195=CARTESIAN_POINT('',(-6.35,23.72275,34.09675)) ;
#8196=CARTESIAN_POINT('',(-6.35,7.4375,33.5)) ;
#8197=CARTESIAN_POINT('Origin',(-9.5,31.75,29.6)) ;
#8198=CARTESIAN_POINT('',(6.325,31.75,29.6)) ;
#8199=CARTESIAN_POINT('',(6.325,35.4862814263725,25.0927398665982)) ;
#8200=CARTESIAN_POINT('',(-6.325,31.75,29.6)) ;
#8201=CARTESIAN_POINT('',(-9.5,31.75,29.6)) ;
#8202=CARTESIAN_POINT('',(-6.325,35.4862814263725,25.0927398665982)) ;
#8203=CARTESIAN_POINT('Origin',(6.325,33.0419144924728,23.0664883292866)) ;
#8204=CARTESIAN_POINT('',(6.8058099585235,28.5460488256182,33.407707310626)) ;
#8205=CARTESIAN_POINT('Origin',(6.325,23.9220039727312,34.0682851467527)) ;
#8206=CARTESIAN_POINT('',(9.5,24.6003192917499,33.25)) ;
#8207=CARTESIAN_POINT('Origin',(6.325,24.6003192917499,33.25)) ;
#8208=CARTESIAN_POINT('',(9.5,28.575,28.4551470821109)) ;
#8209=CARTESIAN_POINT('',(9.5,33.0419144924728,23.0664883292866)) ;
#8210=CARTESIAN_POINT('Origin',(6.325,28.575,28.4551470821109)) ;
#8211=CARTESIAN_POINT('Origin',(-9.5,28.6,33.4)) ;
#8212=CARTESIAN_POINT('',(7.77490213744257,27.9,33.5)) ;
#8213=CARTESIAN_POINT('',(-9.5,27.9,33.5)) ;
#8214=CARTESIAN_POINT('Ctrl Pts',(6.80580995852343,28.5460488256182,33.407707310626)) ;
#8215=CARTESIAN_POINT('Ctrl Pts',(6.98149608419224,28.5063917103341,33.4133726128094)) ;
#8216=CARTESIAN_POINT('Ctrl Pts',(7.15246189889731,28.4448215928176,33.4221683438834)) ;
#8217=CARTESIAN_POINT('Ctrl Pts',(7.51422463753846,28.257594890715,33.4489150156123)) ;
#8218=CARTESIAN_POINT('Ctrl Pts',(7.65963613230187,28.138247635494,33.4659646235008)) ;
#8219=CARTESIAN_POINT('Ctrl Pts',(7.77111347508396,28.0136205242995,33.4837684965286)) ;
#8220=CARTESIAN_POINT('Ctrl Pts',(7.79340206880744,27.9818131636569,33.4883124051919)) ;
#8221=CARTESIAN_POINT('Ctrl Pts',(7.80749608791706,27.9495759565561,33.492917720492)) ;
#8222=CARTESIAN_POINT('Ctrl Pts',(7.81039840242134,27.9412633965255,33.4941052290678)) ;
#8223=CARTESIAN_POINT('Ctrl Pts',(7.81205507027208,27.9288342740703,33.49588081799)) ;
#8224=CARTESIAN_POINT('Ctrl Pts',(7.81211175307097,27.9241339804662,33.4965522885068)) ;
#8225=CARTESIAN_POINT('Ctrl Pts',(7.81035146711017,27.9167681745698,33.497604546492)) ;
#8226=CARTESIAN_POINT('Ctrl Pts',(7.80915473049808,27.9140001175515,33.4979999832069)) ;
#8227=CARTESIAN_POINT('Ctrl Pts',(7.80568132004777,27.9092451830197,33.4986792595686)) ;
#8228=CARTESIAN_POINT('Ctrl Pts',(7.80360341728409,27.907368861679,33.4989473054744)) ;
#8229=CARTESIAN_POINT('Ctrl Pts',(7.79812049420868,27.9038813555221,33.4994455206397)) ;
#8230=CARTESIAN_POINT('Ctrl Pts',(7.79461677020034,27.902571843467,33.4996325937904)) ;
#8231=CARTESIAN_POINT('Ctrl Pts',(7.78586974385829,27.9004243166327,33.4999393833382)) ;
#8232=CARTESIAN_POINT('Ctrl Pts',(7.78023927099663,27.9,33.5)) ;
#8233=CARTESIAN_POINT('Ctrl Pts',(7.77490213744257,27.9,33.5)) ;
#8234=CARTESIAN_POINT('Origin',(-18.25,3.05,10.325)) ;
#8235=CARTESIAN_POINT('',(-18.25,3.3,13.24)) ;
#8236=CARTESIAN_POINT('',(-18.25,3.05,12.99)) ;
#8237=CARTESIAN_POINT('Origin',(-18.25,3.05,13.24)) ;
#8238=CARTESIAN_POINT('',(-18.25,3.05,7.66)) ;
#8239=CARTESIAN_POINT('Origin',(-18.25,3.05,10.325)) ;
#8240=CARTESIAN_POINT('',(-18.25,3.3,7.41)) ;
#8241=CARTESIAN_POINT('Origin',(-18.25,3.05,7.41)) ;
#8242=CARTESIAN_POINT('Origin',(-18.25,3.3,10.325)) ;
#8243=CARTESIAN_POINT('Origin',(-9.12502074844716,3.05,7.41)) ;
#8244=CARTESIAN_POINT('',(-16.75,3.05,7.66)) ;
#8245=CARTESIAN_POINT('',(-16.75,3.3,7.41)) ;
#8246=CARTESIAN_POINT('Origin',(-16.75,3.05,7.41)) ;
#8247=CARTESIAN_POINT('',(-9.12502074844716,3.3,7.41)) ;
#8248=CARTESIAN_POINT('',(-9.12502074844716,3.05,7.66)) ;
#8249=CARTESIAN_POINT('Origin',(-16.75,3.05,10.325)) ;
#8250=CARTESIAN_POINT('',(-16.75,3.05,12.99)) ;
#8251=CARTESIAN_POINT('',(-16.75,3.3,13.24)) ;
#8252=CARTESIAN_POINT('Origin',(-16.75,3.05,13.24)) ;
#8253=CARTESIAN_POINT('Origin',(-16.75,3.3,10.325)) ;
#8254=CARTESIAN_POINT('Origin',(-16.75,3.05,10.325)) ;
#8255=CARTESIAN_POINT('Origin',(-8.37502074844716,3.05,13.24)) ;
#8256=CARTESIAN_POINT('',(-8.37502074844716,3.3,13.24)) ;
#8257=CARTESIAN_POINT('',(-8.37502074844716,3.05,12.99)) ;
#8258=CARTESIAN_POINT('Origin',(-18.25,0.,7.66)) ;
#8259=CARTESIAN_POINT('',(-18.25,0.,7.66)) ;
#8260=CARTESIAN_POINT('',(-18.25,0.,7.66)) ;
#8261=CARTESIAN_POINT('',(-16.75,0.,7.66)) ;
#8262=CARTESIAN_POINT('',(-16.75,0.,7.66)) ;
#8263=CARTESIAN_POINT('',(-16.75,0.,7.66)) ;
#8264=CARTESIAN_POINT('Origin',(-18.25,0.,10.325)) ;
#8265=CARTESIAN_POINT('',(-18.25,0.,12.99)) ;
#8266=CARTESIAN_POINT('',(-18.25,0.,12.99)) ;
#8267=CARTESIAN_POINT('Origin',(-18.25,0.,10.325)) ;
#8268=CARTESIAN_POINT('Origin',(-4.14968943118765E-5,3.3,0.0099999999999989)) ;
#8269=CARTESIAN_POINT('',(-11.5234336016174,3.3,-28.4730130039621)) ;
#8270=CARTESIAN_POINT('',(-10.77,3.3,-29.176932678781)) ;
#8271=CARTESIAN_POINT('Origin',(1.11022302462516E-15,3.3,-16.8941925465839)) ;
#8272=CARTESIAN_POINT('',(-23.6251157417011,3.3,-16.3713308677057)) ;
#8273=CARTESIAN_POINT('',(-15.7632336789269,3.3,-24.2332129304798)) ;
#8274=CARTESIAN_POINT('',(-24.4999998519293,3.3,-14.3009167753159)) ;
#8275=CARTESIAN_POINT('Origin',(-21.664129241231,3.3,-14.3226323462975)) ;
#8276=CARTESIAN_POINT('',(-24.5,3.3,33.25)) ;
#8277=CARTESIAN_POINT('',(-24.5,3.3,-7.145)) ;
#8278=CARTESIAN_POINT('',(-10.77,3.3,33.25)) ;
#8279=CARTESIAN_POINT('',(-12.2500207484472,3.3,33.25)) ;
#8280=CARTESIAN_POINT('',(-10.77,3.3,1.2425)) ;
#8281=CARTESIAN_POINT('',(-18.25,3.3,-8.985)) ;
#8282=CARTESIAN_POINT('Origin',(-18.25,3.3,-11.9)) ;
#8283=CARTESIAN_POINT('Origin',(-18.25,3.05,-11.9)) ;
#8284=CARTESIAN_POINT('',(-18.25,3.05,-9.235)) ;
#8285=CARTESIAN_POINT('Origin',(-18.25,3.05,-8.985)) ;
#8286=CARTESIAN_POINT('',(-20.915,3.05,-11.9)) ;
#8287=CARTESIAN_POINT('Origin',(-18.25,3.05,-11.9)) ;
#8288=CARTESIAN_POINT('Origin',(-18.25,3.05,-11.9)) ;
#8289=CARTESIAN_POINT('Origin',(-18.25,0.,-11.9)) ;
#8290=CARTESIAN_POINT('',(-20.915,0.,-11.9)) ;
#8291=CARTESIAN_POINT('',(-20.915,0.,-11.9)) ;
#8292=CARTESIAN_POINT('Origin',(-18.25,0.,-11.9)) ;
#8293=CARTESIAN_POINT('Origin',(18.25,3.05,-11.9)) ;
#8294=CARTESIAN_POINT('',(18.25,3.3,-8.985)) ;
#8295=CARTESIAN_POINT('Origin',(18.25,3.3,-11.9)) ;
#8296=CARTESIAN_POINT('',(18.25,3.05,-9.235)) ;
#8297=CARTESIAN_POINT('Origin',(18.25,3.05,-8.985)) ;
#8298=CARTESIAN_POINT('',(15.585,3.05,-11.9)) ;
#8299=CARTESIAN_POINT('Origin',(18.25,3.05,-11.9)) ;
#8300=CARTESIAN_POINT('Origin',(18.25,3.05,-11.9)) ;
#8301=CARTESIAN_POINT('Origin',(-4.14968943118765E-5,3.3,0.0099999999999989)) ;
#8302=CARTESIAN_POINT('',(24.5,3.3,33.25)) ;
#8303=CARTESIAN_POINT('',(10.77,3.3,33.25)) ;
#8304=CARTESIAN_POINT('',(-12.2500207484472,3.3,33.25)) ;
#8305=CARTESIAN_POINT('',(24.5,3.3,-14.2973164482764)) ;
#8306=CARTESIAN_POINT('',(24.5,3.3,16.63)) ;
#8307=CARTESIAN_POINT('',(23.6225672795876,3.3,-16.373879130817)) ;
#8308=CARTESIAN_POINT('Origin',(21.4457388066382,3.3,-14.2304230516917)) ;
#8309=CARTESIAN_POINT('',(11.5234336029266,3.3,-28.4730130064801)) ;
#8310=CARTESIAN_POINT('',(21.8132129304798,3.3,-18.1832336789269)) ;
#8311=CARTESIAN_POINT('',(10.77,3.3,-29.176932678781)) ;
#8312=CARTESIAN_POINT('Origin',(1.11022302462516E-15,3.3,-16.8941925465839)) ;
#8313=CARTESIAN_POINT('',(10.77,3.3,1.2425)) ;
#8314=CARTESIAN_POINT('',(16.75,3.3,7.41)) ;
#8315=CARTESIAN_POINT('',(16.75,3.3,13.24)) ;
#8316=CARTESIAN_POINT('Origin',(16.75,3.3,10.325)) ;
#8317=CARTESIAN_POINT('',(18.25,3.3,7.41)) ;
#8318=CARTESIAN_POINT('',(8.37497925155284,3.3,7.41)) ;
#8319=CARTESIAN_POINT('',(18.25,3.3,13.24)) ;
#8320=CARTESIAN_POINT('Origin',(18.25,3.3,10.325)) ;
#8321=CARTESIAN_POINT('',(9.12497925155284,3.3,13.24)) ;
#8322=CARTESIAN_POINT('Origin',(18.25,0.,-11.9)) ;
#8323=CARTESIAN_POINT('',(15.585,0.,-11.9)) ;
#8324=CARTESIAN_POINT('',(15.585,0.,-11.9)) ;
#8325=CARTESIAN_POINT('Origin',(18.25,0.,-11.9)) ;
#8326=CARTESIAN_POINT('Origin',(16.75,3.05,10.325)) ;
#8327=CARTESIAN_POINT('',(16.75,3.05,12.99)) ;
#8328=CARTESIAN_POINT('Origin',(16.75,3.05,13.24)) ;
#8329=CARTESIAN_POINT('',(16.75,3.05,7.66)) ;
#8330=CARTESIAN_POINT('Origin',(16.75,3.05,10.325)) ;
#8331=CARTESIAN_POINT('Origin',(16.75,3.05,7.41)) ;
#8332=CARTESIAN_POINT('Origin',(8.37497925155284,3.05,7.41)) ;
#8333=CARTESIAN_POINT('',(18.25,3.05,7.66)) ;
#8334=CARTESIAN_POINT('Origin',(18.25,3.05,7.41)) ;
#8335=CARTESIAN_POINT('',(8.37497925155284,3.05,7.66)) ;
#8336=CARTESIAN_POINT('Origin',(18.25,3.05,10.325)) ;
#8337=CARTESIAN_POINT('',(18.25,3.05,12.99)) ;
#8338=CARTESIAN_POINT('Origin',(18.25,3.05,13.24)) ;
#8339=CARTESIAN_POINT('Origin',(18.25,3.05,10.325)) ;
#8340=CARTESIAN_POINT('Origin',(9.12497925155284,3.05,13.24)) ;
#8341=CARTESIAN_POINT('',(9.12497925155284,3.05,12.99)) ;
#8342=CARTESIAN_POINT('Origin',(16.75,0.,7.66)) ;
#8343=CARTESIAN_POINT('',(16.75,0.,7.66)) ;
#8344=CARTESIAN_POINT('',(16.75,0.,7.66)) ;
#8345=CARTESIAN_POINT('',(18.25,0.,7.66)) ;
#8346=CARTESIAN_POINT('',(18.25,0.,7.66)) ;
#8347=CARTESIAN_POINT('',(18.25,0.,7.66)) ;
#8348=CARTESIAN_POINT('Origin',(16.75,0.,10.325)) ;
#8349=CARTESIAN_POINT('',(16.75,0.,12.99)) ;
#8350=CARTESIAN_POINT('',(16.75,0.,12.99)) ;
#8351=CARTESIAN_POINT('Origin',(16.75,0.,10.325)) ;
#8352=CARTESIAN_POINT('Ctrl Pts',(6.76795090667119,28.3557987366091,33.5)) ;
#8353=CARTESIAN_POINT('Ctrl Pts',(7.54929504861544,28.2003141923527,33.5)) ;
#8354=CARTESIAN_POINT('Ctrl Pts',(8.81719996776912,27.1694431484449,33.5)) ;
#8355=CARTESIAN_POINT('Ctrl Pts',(9.25,25.370369005669,33.5)) ;
#8356=CARTESIAN_POINT('Ctrl Pts',(9.25,24.6003192917499,33.5)) ;
#8357=CARTESIAN_POINT('Ctrl Pts',(6.77517359820442,28.3920943552222,33.5)) ;
#8358=CARTESIAN_POINT('Ctrl Pts',(7.5693362493457,28.2354900210942,33.5000078650668)) ;
#8359=CARTESIAN_POINT('Ctrl Pts',(8.85942127194598,27.1975612821968,33.4998356946794)) ;
#8360=CARTESIAN_POINT('Ctrl Pts',(9.31001237129095,25.3805985297588,33.4998240176448)) ;
#8361=CARTESIAN_POINT('Ctrl Pts',(9.31544984694979,24.6003192917499,33.5)) ;
#8362=CARTESIAN_POINT('Ctrl Pts',(6.78961185129094,28.464649762726,33.483268532741)) ;
#8363=CARTESIAN_POINT('Ctrl Pts',(7.60938939076488,28.3057987139221,33.4819757476224)) ;
#8364=CARTESIAN_POINT('Ctrl Pts',(8.94398652948134,27.2537008535442,33.4736901555626)) ;
#8365=CARTESIAN_POINT('Ctrl Pts',(9.42982991123221,25.4008861366219,33.4551270066274)) ;
#8366=CARTESIAN_POINT('Ctrl Pts',(9.4456714379219,24.6003192917499,33.4456714379219)) ;
#8367=CARTESIAN_POINT('Ctrl Pts',(6.80125367349468,28.5231524880223,33.4364220663262)) ;
#8368=CARTESIAN_POINT('Ctrl Pts',(7.64149663567339,28.3614500536775,33.4317712233585)) ;
#8369=CARTESIAN_POINT('Ctrl Pts',(9.00760901658297,27.2899950446832,33.4011943379152)) ;
#8370=CARTESIAN_POINT('Ctrl Pts',(9.49134428057035,25.4094606950313,33.342417324315)) ;
#8371=CARTESIAN_POINT('Ctrl Pts',(9.5,24.6003192917499,33.3154498469498)) ;
#8372=CARTESIAN_POINT('Ctrl Pts',(6.80580995852343,28.5460488256182,33.407707310626)) ;
#8373=CARTESIAN_POINT('Ctrl Pts',(7.6539356510612,28.3826875378412,33.4011779048128)) ;
#8374=CARTESIAN_POINT('Ctrl Pts',(9.0302085120229,27.2995932530023,33.3578875866726)) ;
#8375=CARTESIAN_POINT('Ctrl Pts',(9.5,25.4093792116268,33.2823374075703)) ;
#8376=CARTESIAN_POINT('Ctrl Pts',(9.5,24.6003192917499,33.25)) ;
#8377=CARTESIAN_POINT('',(9.25,24.6003192917499,33.5)) ;
#8378=CARTESIAN_POINT('Origin',(6.325,24.6003192917499,33.5)) ;
#8379=CARTESIAN_POINT('Origin',(9.25,24.6003192917499,33.25)) ;
#8380=CARTESIAN_POINT('Origin',(9.25,8.6875,33.25)) ;
#8381=CARTESIAN_POINT('',(9.25,4.57,33.5)) ;
#8382=CARTESIAN_POINT('',(9.5,4.57,33.25)) ;
#8383=CARTESIAN_POINT('Origin',(9.25,4.57,33.25)) ;
#8384=CARTESIAN_POINT('',(9.5,8.6875,33.25)) ;
#8385=CARTESIAN_POINT('',(9.25,8.6875,33.5)) ;
#8386=CARTESIAN_POINT('Origin',(-12.2500207484472,3.05,33.25)) ;
#8387=CARTESIAN_POINT('',(10.77,3.05,33.5)) ;
#8388=CARTESIAN_POINT('Origin',(10.77,3.05,33.25)) ;
#8389=CARTESIAN_POINT('',(24.5,3.05,33.5)) ;
#8390=CARTESIAN_POINT('',(-12.2500207484472,3.05,33.5)) ;
#8391=CARTESIAN_POINT('Origin',(24.5,3.05,33.25)) ;
#8392=CARTESIAN_POINT('Origin',(10.77,4.57,33.25)) ;
#8393=CARTESIAN_POINT('Origin',(10.77,4.57,33.25)) ;
#8394=CARTESIAN_POINT('Origin',(10.77,4.57,33.5)) ;
#8395=CARTESIAN_POINT('Origin',(21.4457388066382,3.05,-14.2304230516917)) ;
#8396=CARTESIAN_POINT('',(24.75,3.05,-14.3)) ;
#8397=CARTESIAN_POINT('',(23.8,3.05,-16.55)) ;
#8398=CARTESIAN_POINT('Origin',(21.4457388066382,3.05,-14.2304230516917)) ;
#8399=CARTESIAN_POINT('Ctrl Pts',(23.8,3.05,-16.55)) ;
#8400=CARTESIAN_POINT('Ctrl Pts',(23.8000293456249,3.06636246173745,-16.5499702155749)) ;
#8401=CARTESIAN_POINT('Ctrl Pts',(23.798910747616,3.08272451888078,-16.5488094001891)) ;
#8402=CARTESIAN_POINT('Ctrl Pts',(23.7966660800154,3.09877258050403,-16.5465393599234)) ;
#8403=CARTESIAN_POINT('Ctrl Pts',(23.7945144670797,3.11415535565185,-16.5443634261687)) ;
#8404=CARTESIAN_POINT('Ctrl Pts',(23.7913285774613,3.12924901836754,-16.5411686882304)) ;
#8405=CARTESIAN_POINT('Ctrl Pts',(23.7871649259446,3.1437876509661,-16.5370110383706)) ;
#8406=CARTESIAN_POINT('Ctrl Pts',(23.7830020587907,3.15832354472801,-16.5328541717429)) ;
#8407=CARTESIAN_POINT('Ctrl Pts',(23.7778619736653,3.17230401141269,-16.5277349297353)) ;
#8408=CARTESIAN_POINT('Ctrl Pts',(23.7718355851639,3.18548283774181,-16.5217430712642)) ;
#8409=CARTESIAN_POINT('Ctrl Pts',(23.765810164708,3.19865954709755,-16.5157521752919)) ;
#8410=CARTESIAN_POINT('Ctrl Pts',(23.7588989785171,3.21103432480559,-16.5088891930629)) ;
#8411=CARTESIAN_POINT('Ctrl Pts',(23.7512241009886,3.22238930539324,-16.5012745467355)) ;
#8412=CARTESIAN_POINT('Ctrl Pts',(23.7435502435946,3.23374277669204,-16.4936609125367)) ;
#8413=CARTESIAN_POINT('Ctrl Pts',(23.7351132191597,3.24407624949196,-16.4852961311533)) ;
#8414=CARTESIAN_POINT('Ctrl Pts',(23.7260619356313,3.25320784483669,-16.4763270162031)) ;
#8415=CARTESIAN_POINT('Ctrl Pts',(23.7170075012856,3.26234261895575,-16.4673547790392)) ;
#8416=CARTESIAN_POINT('Ctrl Pts',(23.7073387574172,3.27027429523935,-16.457778159615)) ;
#8417=CARTESIAN_POINT('Ctrl Pts',(23.6972264211279,3.27686317193747,-16.4477654057518)) ;
#8418=CARTESIAN_POINT('Ctrl Pts',(23.6871172241685,3.28345000314799,-16.4377557603037)) ;
#8419=CARTESIAN_POINT('Ctrl Pts',(23.6765651334693,3.28869459613384,-16.4273106684178)) ;
#8420=CARTESIAN_POINT('Ctrl Pts',(23.6657563222244,3.2925046341702,-16.4166135482745)) ;
#8421=CARTESIAN_POINT('Ctrl Pts',(23.6549466148759,3.29631498807748,-16.4059155412874)) ;
#8422=CARTESIAN_POINT('Ctrl Pts',(23.6438805959438,3.29869038961342,-16.3949659091188)) ;
#8423=CARTESIAN_POINT('Ctrl Pts',(23.6327535307763,3.29958901942994,-16.3839569688262)) ;
#8424=CARTESIAN_POINT('Ctrl Pts',(23.6293618826288,3.29986293138305,-16.3806013264006)) ;
#8425=CARTESIAN_POINT('Ctrl Pts',(23.625964600032,3.3,-16.3772402100488)) ;
#8426=CARTESIAN_POINT('Ctrl Pts',(23.6225672795876,3.3,-16.373879130817)) ;
#8427=CARTESIAN_POINT('Ctrl Pts',(24.5,3.3,-14.2973164482764)) ;
#8428=CARTESIAN_POINT('Ctrl Pts',(24.5015396345052,3.3,-14.2973333065323)) ;
#8429=CARTESIAN_POINT('Ctrl Pts',(24.5030792362479,3.29998577715355,-14.297350158057)) ;
#8430=CARTESIAN_POINT('Ctrl Pts',(24.5367196937611,3.29936418270175,-14.2977182266959)) ;
#8431=CARTESIAN_POINT('Ctrl Pts',(24.5684081693065,3.29259261132557,-14.2980620867652)) ;
#8432=CARTESIAN_POINT('Ctrl Pts',(24.6278990054925,3.26725920437385,-14.2987032837107)) ;
#8433=CARTESIAN_POINT('Ctrl Pts',(24.6550726110038,3.24877687466915,-14.2989938308607)) ;
#8434=CARTESIAN_POINT('Ctrl Pts',(24.7008047506126,3.20243716760779,-14.2994805987249)) ;
#8435=CARTESIAN_POINT('Ctrl Pts',(24.7189265638722,3.17502334972294,-14.2996722340112)) ;
#8436=CARTESIAN_POINT('Ctrl Pts',(24.7436421992149,3.11479271760787,-14.2999331603654)) ;
#8437=CARTESIAN_POINT('Ctrl Pts',(24.75,3.08255201651694,-14.3)) ;
#8438=CARTESIAN_POINT('Ctrl Pts',(24.75,3.05,-14.3)) ;
#8439=CARTESIAN_POINT('Origin',(-21.664129241231,3.05,-14.3226323462975)) ;
#8440=CARTESIAN_POINT('',(-24.75,3.05,-14.3)) ;
#8441=CARTESIAN_POINT('Ctrl Pts',(-24.75,3.05,-14.3)) ;
#8442=CARTESIAN_POINT('Ctrl Pts',(-24.7499996951622,3.06636246173745,-14.2999584360325)) ;
#8443=CARTESIAN_POINT('Ctrl Pts',(-24.7483879108569,3.08272451888078,-14.2999286913692)) ;
#8444=CARTESIAN_POINT('Ctrl Pts',(-24.745195533686,3.09877258050403,-14.2999107323432)) ;
#8445=CARTESIAN_POINT('Ctrl Pts',(-24.7421354993356,3.11415535553231,-14.2998935178246)) ;
#8446=CARTESIAN_POINT('Ctrl Pts',(-24.7376237166988,3.12924901813298,-14.2998871289039)) ;
#8447=CARTESIAN_POINT('Ctrl Pts',(-24.7317396696698,3.14378765062717,-14.2998911419599)) ;
#8448=CARTESIAN_POINT('Ctrl Pts',(-24.7258567310994,3.15832354427998,-14.2998951542599)) ;
#8449=CARTESIAN_POINT('Ctrl Pts',(-24.7186022921447,3.17230401086657,-14.2999095634098)) ;
#8450=CARTESIAN_POINT('Ctrl Pts',(-24.7101041084036,3.18548283711434,-14.299933571763)) ;
#8451=CARTESIAN_POINT('Ctrl Pts',(-24.7016072897667,3.19865954638359,-14.2999575762596)) ;
#8452=CARTESIAN_POINT('Ctrl Pts',(-24.6918674814275,3.21103432402251,-14.2999911747909)) ;
#8453=CARTESIAN_POINT('Ctrl Pts',(-24.6810561544944,3.22238930456332,-14.3000332206547)) ;
#8454=CARTESIAN_POINT('Ctrl Pts',(-24.6702462645928,3.23374277581057,-14.3000752609299)) ;
#8455=CARTESIAN_POINT('Ctrl Pts',(-24.6583655923458,3.24407624858209,-14.3001257433967)) ;
#8456=CARTESIAN_POINT('Ctrl Pts',(-24.6456232446371,3.25320784392526,-14.3001832098595)) ;
#8457=CARTESIAN_POINT('Ctrl Pts',(-24.6328764612318,3.26234261803794,-14.3002406963268)) ;
#8458=CARTESIAN_POINT('Ctrl Pts',(-24.6192679322756,3.27027429434331,-14.300305168057)) ;
#8459=CARTESIAN_POINT('Ctrl Pts',(-24.6050373423276,3.27686317109361,-14.3003749019062)) ;
#8460=CARTESIAN_POINT('Ctrl Pts',(-24.590811170207,3.28345000235455,-14.3004446141069)) ;
#8461=CARTESIAN_POINT('Ctrl Pts',(-24.5759639176278,3.28869459542192,-14.300519580942)) ;
#8462=CARTESIAN_POINT('Ctrl Pts',(-24.5607569253176,3.29250463357125,-14.3005978764304)) ;
#8463=CARTESIAN_POINT('Ctrl Pts',(-24.5455486722758,3.29631498759076,-14.3006761784098)) ;
#8464=CARTESIAN_POINT('Ctrl Pts',(-24.529981253701,3.29869038927096,-14.3007578049366)) ;
#8465=CARTESIAN_POINT('Ctrl Pts',(-24.514328731891,3.29958901926202,-14.3008406917336)) ;
#8466=CARTESIAN_POINT('Ctrl Pts',(-24.5095576752671,3.29986293132702,-14.3008659565189)) ;
#8467=CARTESIAN_POINT('Ctrl Pts',(-24.5047787638457,3.3,-14.3008913376992)) ;
#8468=CARTESIAN_POINT('Ctrl Pts',(-24.4999998519293,3.3,-14.3009167753159)) ;
#8469=CARTESIAN_POINT('',(-23.8,3.05,-16.55)) ;
#8470=CARTESIAN_POINT('Ctrl Pts',(-23.6251157417011,3.3,-16.3713308677057)) ;
#8471=CARTESIAN_POINT('Ctrl Pts',(-23.6262285835138,3.3,-16.372468319203)) ;
#8472=CARTESIAN_POINT('Ctrl Pts',(-23.6273414052155,3.29998480854004,-16.3736057396723)) ;
#8473=CARTESIAN_POINT('Ctrl Pts',(-23.6508682580149,3.29934240875891,-16.3976524294703)) ;
#8474=CARTESIAN_POINT('Ctrl Pts',(-23.6729946612897,3.29257223359693,-16.4202633562148)) ;
#8475=CARTESIAN_POINT('Ctrl Pts',(-23.7145752356494,3.26725923592507,-16.4627478051389)) ;
#8476=CARTESIAN_POINT('Ctrl Pts',(-23.7335850472872,3.24877691508736,-16.4821672771834)) ;
#8477=CARTESIAN_POINT('Ctrl Pts',(-23.7655795153817,3.2024372164242,-16.5148478457573)) ;
#8478=CARTESIAN_POINT('Ctrl Pts',(-23.7782585885107,3.17502339467209,-16.527796901805)) ;
#8479=CARTESIAN_POINT('Ctrl Pts',(-23.795551415589,3.11479274608981,-16.5454572885827)) ;
#8480=CARTESIAN_POINT('Ctrl Pts',(-23.7999999999999,3.0825520303151,-16.5500000000001)) ;
#8481=CARTESIAN_POINT('Ctrl Pts',(-23.7999999999999,3.05,-16.5500000000001)) ;
#8482=CARTESIAN_POINT('Origin',(-21.664129241231,3.05,-14.3226323462975)) ;
#8483=CARTESIAN_POINT('Origin',(-15.7632336789269,3.05,-24.2332129304798)) ;
#8484=CARTESIAN_POINT('',(-11.7,3.05,-28.65)) ;
#8485=CARTESIAN_POINT('Ctrl Pts',(-11.5234344017198,3.3,-28.473012207687)) ;
#8486=CARTESIAN_POINT('Ctrl Pts',(-11.5248174913711,3.3,-28.4743986171271)) ;
#8487=CARTESIAN_POINT('Ctrl Pts',(-11.5262005335124,3.29997698962268,-28.4757849786368)) ;
#8488=CARTESIAN_POINT('Ctrl Pts',(-11.549952120929,3.29918654602524,-28.4995935660478)) ;
#8489=CARTESIAN_POINT('Ctrl Pts',(-11.5720185826081,3.29242837602069,-28.5217129029688)) ;
#8490=CARTESIAN_POINT('Ctrl Pts',(-11.6137589203919,3.26726387118117,-28.5635531294894)) ;
#8491=CARTESIAN_POINT('Ctrl Pts',(-11.6329511205585,3.24878239907981,-28.5827911879915)) ;
#8492=CARTESIAN_POINT('Ctrl Pts',(-11.6652519474713,3.2024434132778,-28.6151691262904)) ;
#8493=CARTESIAN_POINT('Ctrl Pts',(-11.6780517643173,3.17502893211547,-28.62799946099)) ;
#8494=CARTESIAN_POINT('Ctrl Pts',(-11.6955092411612,3.11479613681779,-28.6454985466271)) ;
#8495=CARTESIAN_POINT('Ctrl Pts',(-11.7,3.08255368454758,-28.65)) ;
#8496=CARTESIAN_POINT('Ctrl Pts',(-11.7,3.05,-28.65)) ;
#8497=CARTESIAN_POINT('',(-15.9400103742236,3.05,-24.4099896257764)) ;
#8498=CARTESIAN_POINT('Ctrl Pts',(10.4512438343541,3.34065281272427,-29.501243923759)) ;
#8499=CARTESIAN_POINT('Ctrl Pts',(10.5574497695917,3.31311478519587,-29.3965002427796)) ;
#8500=CARTESIAN_POINT('Ctrl Pts',(10.6644750033045,3.3,-29.2876755180677)) ;
#8501=CARTESIAN_POINT('Ctrl Pts',(10.77,3.3,-29.176932678781)) ;
#8502=CARTESIAN_POINT('Ctrl Pts',(10.4867185411393,3.33145461255,-29.5471888940564)) ;
#8503=CARTESIAN_POINT('Ctrl Pts',(10.5959487962567,3.30645872447267,-29.4433768078905)) ;
#8504=CARTESIAN_POINT('Ctrl Pts',(10.7056436255396,3.29633423430578,-29.3355995974396)) ;
#8505=CARTESIAN_POINT('Ctrl Pts',(10.8131502913865,3.3,-29.2261438037327)) ;
#8506=CARTESIAN_POINT('Ctrl Pts',(10.5465724667282,3.27117973026827,-29.6387913916651)) ;
#8507=CARTESIAN_POINT('Ctrl Pts',(10.6646000202358,3.24691483243654,-29.5367571598192)) ;
#8508=CARTESIAN_POINT('Ctrl Pts',(10.7830438290637,3.2389968774968,-29.4311063020666)) ;
#8509=CARTESIAN_POINT('Ctrl Pts',(10.8990265225851,3.24570588944608,-29.3240820981936)) ;
#8510=CARTESIAN_POINT('Ctrl Pts',(10.5563795789494,3.15628364564047,-29.6868463778552)) ;
#8511=CARTESIAN_POINT('Ctrl Pts',(10.6826104679429,3.12626473336083,-29.5827439357331)) ;
#8512=CARTESIAN_POINT('Ctrl Pts',(10.8096178153565,3.11314703296705,-29.4745902410339)) ;
#8513=CARTESIAN_POINT('Ctrl Pts',(10.9348219720805,3.11544984694979,-29.3649053297691)) ;
#8514=CARTESIAN_POINT('Ctrl Pts',(10.5474800757194,3.09865533491409,-29.6941797705656)) ;
#8515=CARTESIAN_POINT('Ctrl Pts',(10.6765379977093,3.06569643582498,-29.587833112793)) ;
#8516=CARTESIAN_POINT('Ctrl Pts',(10.8065915039711,3.05,-29.4773429557935)) ;
#8517=CARTESIAN_POINT('Ctrl Pts',(10.9348219720805,3.05,-29.3649053297691)) ;
#8518=CARTESIAN_POINT('',(10.4512438329193,3.34065280720824,-29.5012439237535)) ;
#8519=CARTESIAN_POINT('Ctrl Pts',(10.4512438343541,3.34065281272427,-29.501243923759)) ;
#8520=CARTESIAN_POINT('Ctrl Pts',(10.5574497695917,3.31311478519587,-29.3965002427796)) ;
#8521=CARTESIAN_POINT('Ctrl Pts',(10.6644750033045,3.3,-29.2876755180677)) ;
#8522=CARTESIAN_POINT('Ctrl Pts',(10.77,3.3,-29.176932678781)) ;
#8523=CARTESIAN_POINT('',(10.9348219720805,3.05,-29.3649053297691)) ;
#8524=CARTESIAN_POINT('Origin',(10.77,3.05,-29.176932678781)) ;
#8525=CARTESIAN_POINT('',(10.5823632225196,3.09017244597965,-29.6653552778491)) ;
#8526=CARTESIAN_POINT('Ctrl Pts',(10.9348219720805,3.05,-29.3649053297691)) ;
#8527=CARTESIAN_POINT('Ctrl Pts',(10.8181371295453,3.05,-29.4672192874511)) ;
#8528=CARTESIAN_POINT('Ctrl Pts',(10.6999427554713,3.06299713058315,-29.5679206810131)) ;
#8529=CARTESIAN_POINT('Ctrl Pts',(10.5823626153175,3.09017135645643,-29.6653548535384)) ;
#8530=CARTESIAN_POINT('',(10.4562560925639,3.33923511979837,-29.5067623750852)) ;
#8531=CARTESIAN_POINT('Ctrl Pts',(10.5823613854325,3.09017164069861,-29.6653558726971)) ;
#8532=CARTESIAN_POINT('Ctrl Pts',(10.5823677899508,3.09071784580571,-29.6653506827371)) ;
#8533=CARTESIAN_POINT('Ctrl Pts',(10.5823730307843,3.09126403335751,-29.6653440861951)) ;
#8534=CARTESIAN_POINT('Ctrl Pts',(10.5823771106453,3.09181019549258,-29.6653360863522)) ;
#8535=CARTESIAN_POINT('Ctrl Pts',(10.5824953065254,3.10763282149373,-29.6651043263781)) ;
#8536=CARTESIAN_POINT('Ctrl Pts',(10.581641197747,3.12338319864702,-29.6636993620564)) ;
#8537=CARTESIAN_POINT('Ctrl Pts',(10.5798821820818,3.13887085021686,-29.6612010522168)) ;
#8538=CARTESIAN_POINT('Ctrl Pts',(10.5788028689804,3.14837390671523,-29.6596681161581)) ;
#8539=CARTESIAN_POINT('Ctrl Pts',(10.5773821081474,3.15777816572057,-29.6577227554171)) ;
#8540=CARTESIAN_POINT('Ctrl Pts',(10.5756284659994,3.16703794902945,-29.6553769789403)) ;
#8541=CARTESIAN_POINT('Ctrl Pts',(10.5727717533484,3.18212229229376,-29.6515556694758)) ;
#8542=CARTESIAN_POINT('Ctrl Pts',(10.5690518851304,3.19672783154786,-29.6466977551295)) ;
#8543=CARTESIAN_POINT('Ctrl Pts',(10.5645156102124,3.21065867009823,-29.640864699056)) ;
#8544=CARTESIAN_POINT('Ctrl Pts',(10.5617795259203,3.21906114773045,-29.6373464526124)) ;
#8545=CARTESIAN_POINT('Ctrl Pts',(10.5587457101495,3.22721796960851,-29.6334728036728)) ;
#8546=CARTESIAN_POINT('Ctrl Pts',(10.5554180283936,3.23508172139697,-29.629252267027)) ;
#8547=CARTESIAN_POINT('Ctrl Pts',(10.5525046602579,3.24196639534373,-29.6255572090613)) ;
#8548=CARTESIAN_POINT('Ctrl Pts',(10.54937781422,3.24859840739661,-29.6216111610704)) ;
#8549=CARTESIAN_POINT('Ctrl Pts',(10.5460432855329,3.2549488825252,-29.6174233243881)) ;
#8550=CARTESIAN_POINT('Ctrl Pts',(10.5397549905257,3.26692468624192,-29.6095258507203)) ;
#8551=CARTESIAN_POINT('Ctrl Pts',(10.5327298507231,3.27790178281476,-29.600769706281)) ;
#8552=CARTESIAN_POINT('Ctrl Pts',(10.5250883209327,3.28777924334128,-29.5912904807446)) ;
#8553=CARTESIAN_POINT('Ctrl Pts',(10.5209275848499,3.29315742121225,-29.5861291378187)) ;
#8554=CARTESIAN_POINT('Ctrl Pts',(10.5165835641967,3.29820896154503,-29.5807530157848)) ;
#8555=CARTESIAN_POINT('Ctrl Pts',(10.5120725594015,3.30291220128229,-29.5751821384144)) ;
#8556=CARTESIAN_POINT('Ctrl Pts',(10.5036194939666,3.31172549123882,-29.5647430027716)) ;
#8557=CARTESIAN_POINT('Ctrl Pts',(10.4946636079744,3.31923399426322,-29.5537197514597)) ;
#8558=CARTESIAN_POINT('Ctrl Pts',(10.4853242585872,3.32533098308598,-29.5422670754818)) ;
#8559=CARTESIAN_POINT('Ctrl Pts',(10.4759849091999,3.33142797190874,-29.530814399504)) ;
#8560=CARTESIAN_POINT('Ctrl Pts',(10.4662611466213,3.33611439356466,-29.5189310532188)) ;
#8561=CARTESIAN_POINT('Ctrl Pts',(10.4562542977309,3.33923061889938,-29.506761629053)) ;
#8562=CARTESIAN_POINT('Ctrl Pts',(10.4562560925639,3.33923511979837,-29.5067623750852)) ;
#8563=CARTESIAN_POINT('Ctrl Pts',(10.454686244446,3.33972076841164,-29.5048541775706)) ;
#8564=CARTESIAN_POINT('Ctrl Pts',(10.4530149306185,3.34019358706778,-29.5030149306185)) ;
#8565=CARTESIAN_POINT('Ctrl Pts',(10.4512438793665,3.34065280105307,-29.5012438793665)) ;
#8566=CARTESIAN_POINT('Ctrl Pts',(-10.4562560925639,3.33923511979837,-29.5067623750852)) ;
#8567=CARTESIAN_POINT('Ctrl Pts',(-10.3042079931798,3.31229863060029,-29.6126005064717)) ;
#8568=CARTESIAN_POINT('Ctrl Pts',(-10.1477491130449,3.3,-29.7175603525465)) ;
#8569=CARTESIAN_POINT('Ctrl Pts',(-9.98909940046129,3.3,-29.8200000000001)) ;
#8570=CARTESIAN_POINT('Ctrl Pts',(-10.4937439232518,3.32847961370675,-29.5490226213438)) ;
#8571=CARTESIAN_POINT('Ctrl Pts',(-10.3424189419941,3.3045346571375,-29.6585580134996)) ;
#8572=CARTESIAN_POINT('Ctrl Pts',(-10.1867667904971,3.29572909993472,-29.7667751370844)) ;
#8573=CARTESIAN_POINT('Ctrl Pts',(-10.0291209928307,3.3,-29.8717875912741)) ;
#8574=CARTESIAN_POINT('Ctrl Pts',(-10.5685054554551,3.2669079755233,-29.62309040069)) ;
#8575=CARTESIAN_POINT('Ctrl Pts',(-10.418549761391,3.24402514762918,-29.742418677397)) ;
#8576=CARTESIAN_POINT('Ctrl Pts',(-10.2645399752037,3.23788937883,-29.8603708829999)) ;
#8577=CARTESIAN_POINT('Ctrl Pts',(-10.1087705983175,3.24570589574959,-29.9748534857045)) ;
#8578=CARTESIAN_POINT('Ctrl Pts',(-10.6091727180391,3.15371643721036,-29.6430963665886)) ;
#8579=CARTESIAN_POINT('Ctrl Pts',(-10.4570254125938,3.1246417608215,-29.7697804551427)) ;
#8580=CARTESIAN_POINT('Ctrl Pts',(-10.3004417599091,3.11276689086104,-29.8952373576481)) ;
#8581=CARTESIAN_POINT('Ctrl Pts',(-10.1419706226055,3.11544984694979,-30.01781402741)) ;
#8582=CARTESIAN_POINT('Ctrl Pts',(-10.6162765892914,3.09695856857757,-29.6371780782973)) ;
#8583=CARTESIAN_POINT('Ctrl Pts',(-10.4619015755534,3.06471962087594,-29.7657890572739)) ;
#8584=CARTESIAN_POINT('Ctrl Pts',(-10.3030482793393,3.05,-29.8933327731359)) ;
#8585=CARTESIAN_POINT('Ctrl Pts',(-10.1419706226054,3.05,-30.01781402741)) ;
#8586=CARTESIAN_POINT('',(-10.4562560925639,3.33923511979837,-29.5067623750852)) ;
#8587=CARTESIAN_POINT('',(-9.9890994004613,3.3,-29.82)) ;
#8588=CARTESIAN_POINT('Ctrl Pts',(-10.4562560925639,3.33923511979837,-29.5067623750852)) ;
#8589=CARTESIAN_POINT('Ctrl Pts',(-10.3042079931798,3.31229863060029,-29.6126005064717)) ;
#8590=CARTESIAN_POINT('Ctrl Pts',(-10.1477491130449,3.3,-29.7175603525465)) ;
#8591=CARTESIAN_POINT('Ctrl Pts',(-9.98909940046129,3.3,-29.8200000000001)) ;
#8592=CARTESIAN_POINT('',(-10.1419706226054,3.05,-30.01781402741)) ;
#8593=CARTESIAN_POINT('Origin',(-9.98909940046129,3.05,-29.8200000000001)) ;
#8594=CARTESIAN_POINT('',(-10.5823632225197,3.09017244597965,-29.6653552778491)) ;
#8595=CARTESIAN_POINT('Ctrl Pts',(-10.1419706226054,3.05,-30.01781402741)) ;
#8596=CARTESIAN_POINT('Ctrl Pts',(-10.2912776199237,3.05,-29.902429170969)) ;
#8597=CARTESIAN_POINT('Ctrl Pts',(-10.4386734667128,3.06264696571335,-29.7844130751078)) ;
#8598=CARTESIAN_POINT('Ctrl Pts',(-10.582363125788,3.09017060002378,-29.6653547280519)) ;
#8599=CARTESIAN_POINT('Ctrl Pts',(-10.5823645492884,3.0901708726946,-29.6653535485681)) ;
#8600=CARTESIAN_POINT('Ctrl Pts',(-10.58237093712,3.09071707945032,-29.6653483728594)) ;
#8601=CARTESIAN_POINT('Ctrl Pts',(-10.5823761674002,3.09126326962449,-29.6653417898471)) ;
#8602=CARTESIAN_POINT('Ctrl Pts',(-10.5823802426207,3.09180943533062,-29.6653338028838)) ;
#8603=CARTESIAN_POINT('Ctrl Pts',(-10.5824983793995,3.10764226162414,-29.6651022683863)) ;
#8604=CARTESIAN_POINT('Ctrl Pts',(-10.5816487421359,3.12340351212708,-29.6636948191982)) ;
#8605=CARTESIAN_POINT('Ctrl Pts',(-10.5798917143156,3.13890174174782,-29.661194637388)) ;
#8606=CARTESIAN_POINT('Ctrl Pts',(-10.5788154289346,3.14839534098403,-29.6596631254215)) ;
#8607=CARTESIAN_POINT('Ctrl Pts',(-10.5773980105714,3.15779035973712,-29.6577207127312)) ;
#8608=CARTESIAN_POINT('Ctrl Pts',(-10.575648075692,3.16704107189944,-29.6553786680892)) ;
#8609=CARTESIAN_POINT('Ctrl Pts',(-10.572793572054,3.18213088571561,-29.6515583116694)) ;
#8610=CARTESIAN_POINT('Ctrl Pts',(-10.5690737974298,3.1967412659164,-29.6467011743094)) ;
#8611=CARTESIAN_POINT('Ctrl Pts',(-10.5645335593023,3.21067545103312,-29.6408676243673)) ;
#8612=CARTESIAN_POINT('Ctrl Pts',(-10.5617972837458,3.21907319781733,-29.6373519056613)) ;
#8613=CARTESIAN_POINT('Ctrl Pts',(-10.5587624736304,3.22722513283465,-29.6334807311337)) ;
#8614=CARTESIAN_POINT('Ctrl Pts',(-10.5554349224176,3.23508368100507,-29.6292603598437)) ;
#8615=CARTESIAN_POINT('Ctrl Pts',(-10.5529664611125,3.24091334998174,-29.6261295821166)) ;
#8616=CARTESIAN_POINT('Ctrl Pts',(-10.5503452912355,3.24656143395102,-29.6228172996488)) ;
#8617=CARTESIAN_POINT('Ctrl Pts',(-10.5475756406467,3.25201040996413,-29.6193284766451)) ;
#8618=CARTESIAN_POINT('Ctrl Pts',(-10.541406136158,3.26414821612172,-29.6115569876104)) ;
#8619=CARTESIAN_POINT('Ctrl Pts',(-10.5345010451408,3.27530068412359,-29.6029117174434)) ;
#8620=CARTESIAN_POINT('Ctrl Pts',(-10.5269668631543,3.28536494341284,-29.5935395852846)) ;
#8621=CARTESIAN_POINT('Ctrl Pts',(-10.5222573308481,3.29165599854599,-29.5876811710256)) ;
#8622=CARTESIAN_POINT('Ctrl Pts',(-10.5173015595218,3.29752119279001,-29.5815380059231)) ;
#8623=CARTESIAN_POINT('Ctrl Pts',(-10.5121231599117,3.30292691930815,-29.5751405663713)) ;
#8624=CARTESIAN_POINT('Ctrl Pts',(-10.5036737279875,3.31174727340488,-29.5647020652798)) ;
#8625=CARTESIAN_POINT('Ctrl Pts',(-10.494711970624,3.31926224841926,-29.5536886810406)) ;
#8626=CARTESIAN_POINT('Ctrl Pts',(-10.4853613533682,3.32535947250976,-29.5422471616422)) ;
#8627=CARTESIAN_POINT('Ctrl Pts',(-10.4760107361123,3.33145669660025,-29.5308056422437)) ;
#8628=CARTESIAN_POINT('Ctrl Pts',(-10.4662702167324,3.33613714779707,-29.5189348436387)) ;
#8629=CARTESIAN_POINT('Ctrl Pts',(-10.4562560925639,3.33923511979837,-29.5067623750852)) ;
#8630=CARTESIAN_POINT('Origin',(1.11022302462516E-15,3.05,-16.8941925465839)) ;
#8631=CARTESIAN_POINT('',(9.98909940046138,3.3,-29.82)) ;
#8632=CARTESIAN_POINT('',(10.1419706226055,3.05,-30.01781402741)) ;
#8633=CARTESIAN_POINT('Origin',(9.98909940046138,3.05,-29.82)) ;
#8634=CARTESIAN_POINT('Origin',(1.11022302462516E-15,3.05,-16.8941925465839)) ;
#8635=CARTESIAN_POINT('Origin',(1.11022302462516E-15,3.3,-16.8941925465839)) ;
#8636=CARTESIAN_POINT('Ctrl Pts',(9.98909940046138,3.3,-29.82)) ;
#8637=CARTESIAN_POINT('Ctrl Pts',(10.147749113045,3.3,-29.7175603525465)) ;
#8638=CARTESIAN_POINT('Ctrl Pts',(10.3042079931798,3.3122986306003,-29.6126005064717)) ;
#8639=CARTESIAN_POINT('Ctrl Pts',(10.4562560925639,3.33923511979837,-29.5067623750852)) ;
#8640=CARTESIAN_POINT('Ctrl Pts',(10.0291209928308,3.3,-29.871787591274)) ;
#8641=CARTESIAN_POINT('Ctrl Pts',(10.1867667904972,3.29572909993472,-29.7667751370844)) ;
#8642=CARTESIAN_POINT('Ctrl Pts',(10.3424189419942,3.30453465713751,-29.6585580134996)) ;
#8643=CARTESIAN_POINT('Ctrl Pts',(10.4937439232518,3.32847961370676,-29.5490226213438)) ;
#8644=CARTESIAN_POINT('Ctrl Pts',(10.1087705983176,3.24570589574959,-29.9748534857044)) ;
#8645=CARTESIAN_POINT('Ctrl Pts',(10.2645399752038,3.23788937883,-29.8603708829999)) ;
#8646=CARTESIAN_POINT('Ctrl Pts',(10.4185497613911,3.24402514762919,-29.742418677397)) ;
#8647=CARTESIAN_POINT('Ctrl Pts',(10.5685054554551,3.2669079755233,-29.62309040069)) ;
#8648=CARTESIAN_POINT('Ctrl Pts',(10.1419706226055,3.11544984694979,-30.01781402741)) ;
#8649=CARTESIAN_POINT('Ctrl Pts',(10.3004417599092,3.11276689086104,-29.895237357648)) ;
#8650=CARTESIAN_POINT('Ctrl Pts',(10.4570254125938,3.12464176082151,-29.7697804551426)) ;
#8651=CARTESIAN_POINT('Ctrl Pts',(10.6091727180391,3.15371643721036,-29.6430963665886)) ;
#8652=CARTESIAN_POINT('Ctrl Pts',(10.1419706226055,3.05,-30.01781402741)) ;
#8653=CARTESIAN_POINT('Ctrl Pts',(10.3030482793393,3.05,-29.8933327731359)) ;
#8654=CARTESIAN_POINT('Ctrl Pts',(10.4619015755534,3.06471962087595,-29.7657890572739)) ;
#8655=CARTESIAN_POINT('Ctrl Pts',(10.6162765892914,3.09695856857757,-29.6371780782973)) ;
#8656=CARTESIAN_POINT('Ctrl Pts',(10.582363125788,3.09017060002378,-29.6653547280519)) ;
#8657=CARTESIAN_POINT('Ctrl Pts',(10.4386734667128,3.06264696571336,-29.7844130751078)) ;
#8658=CARTESIAN_POINT('Ctrl Pts',(10.2912776199237,3.05,-29.902429170969)) ;
#8659=CARTESIAN_POINT('Ctrl Pts',(10.1419706226055,3.05,-30.01781402741)) ;
#8660=CARTESIAN_POINT('Ctrl Pts',(9.98909940046138,3.3,-29.82)) ;
#8661=CARTESIAN_POINT('Ctrl Pts',(10.147749113045,3.3,-29.7175603525465)) ;
#8662=CARTESIAN_POINT('Ctrl Pts',(10.3042079931798,3.3122986306003,-29.6126005064717)) ;
#8663=CARTESIAN_POINT('Ctrl Pts',(10.4562560925639,3.33923511979837,-29.5067623750852)) ;
#8664=CARTESIAN_POINT('Origin',(1.11022302462516E-15,3.05,-16.8941925465839)) ;
#8665=CARTESIAN_POINT('',(-10.9348219720805,3.05,-29.3649053297691)) ;
#8666=CARTESIAN_POINT('Origin',(-10.77,3.05,-29.176932678781)) ;
#8667=CARTESIAN_POINT('Origin',(1.11022302462516E-15,3.05,-16.8941925465839)) ;
#8668=CARTESIAN_POINT('Ctrl Pts',(-10.77,3.3,-29.176932678781)) ;
#8669=CARTESIAN_POINT('Ctrl Pts',(-10.6644750033044,3.3,-29.2876755180678)) ;
#8670=CARTESIAN_POINT('Ctrl Pts',(-10.5574497695917,3.31311478519588,-29.3965002427796)) ;
#8671=CARTESIAN_POINT('Ctrl Pts',(-10.4512438343541,3.34065281272427,-29.501243923759)) ;
#8672=CARTESIAN_POINT('Ctrl Pts',(-10.8131502913865,3.3,-29.2261438037327)) ;
#8673=CARTESIAN_POINT('Ctrl Pts',(-10.7056436255395,3.29633423430578,-29.3355995974397)) ;
#8674=CARTESIAN_POINT('Ctrl Pts',(-10.5959487962567,3.30645872447267,-29.4433768078905)) ;
#8675=CARTESIAN_POINT('Ctrl Pts',(-10.4867185411393,3.33145461255,-29.5471888940564)) ;
#8676=CARTESIAN_POINT('Ctrl Pts',(-10.8990265225851,3.24570588944608,-29.3240820981936)) ;
#8677=CARTESIAN_POINT('Ctrl Pts',(-10.7830438290636,3.2389968774968,-29.4311063020667)) ;
#8678=CARTESIAN_POINT('Ctrl Pts',(-10.6646000202357,3.24691483243654,-29.5367571598192)) ;
#8679=CARTESIAN_POINT('Ctrl Pts',(-10.5465724667282,3.27117973026827,-29.6387913916651)) ;
#8680=CARTESIAN_POINT('Ctrl Pts',(-10.9348219720805,3.11544984694979,-29.3649053297691)) ;
#8681=CARTESIAN_POINT('Ctrl Pts',(-10.8096178153564,3.11314703296704,-29.474590241034)) ;
#8682=CARTESIAN_POINT('Ctrl Pts',(-10.6826104679429,3.12626473336083,-29.5827439357331)) ;
#8683=CARTESIAN_POINT('Ctrl Pts',(-10.5563795789494,3.15628364564047,-29.6868463778552)) ;
#8684=CARTESIAN_POINT('Ctrl Pts',(-10.9348219720805,3.05,-29.3649053297691)) ;
#8685=CARTESIAN_POINT('Ctrl Pts',(-10.8065915039709,3.05,-29.4773429557936)) ;
#8686=CARTESIAN_POINT('Ctrl Pts',(-10.6765379977093,3.06569643582498,-29.587833112793)) ;
#8687=CARTESIAN_POINT('Ctrl Pts',(-10.5474800757194,3.09865533491409,-29.6941797705656)) ;
#8688=CARTESIAN_POINT('Ctrl Pts',(-10.5823626153175,3.09017135645643,-29.6653548535384)) ;
#8689=CARTESIAN_POINT('Ctrl Pts',(-10.6999427554713,3.06299713058314,-29.5679206810131)) ;
#8690=CARTESIAN_POINT('Ctrl Pts',(-10.8181371295452,3.05,-29.4672192874512)) ;
#8691=CARTESIAN_POINT('Ctrl Pts',(-10.9348219720805,3.05,-29.3649053297691)) ;
#8692=CARTESIAN_POINT('',(-10.4512438329193,3.34065280720824,-29.5012439237535)) ;
#8693=CARTESIAN_POINT('Ctrl Pts',(-10.77,3.3,-29.176932678781)) ;
#8694=CARTESIAN_POINT('Ctrl Pts',(-10.6644750033044,3.3,-29.2876755180678)) ;
#8695=CARTESIAN_POINT('Ctrl Pts',(-10.5574497695917,3.31311478519588,-29.3965002427796)) ;
#8696=CARTESIAN_POINT('Ctrl Pts',(-10.4512438343541,3.34065281272427,-29.501243923759)) ;
#8697=CARTESIAN_POINT('Ctrl Pts',(-10.4512438793665,3.34065280105307,-29.5012438793665)) ;
#8698=CARTESIAN_POINT('Ctrl Pts',(-10.4530174819393,3.34019292553853,-29.5030174819393)) ;
#8699=CARTESIAN_POINT('Ctrl Pts',(-10.4546884899342,3.33972007374684,-29.504856907029)) ;
#8700=CARTESIAN_POINT('Ctrl Pts',(-10.4562560925639,3.33923511979837,-29.5067623750852)) ;
#8701=CARTESIAN_POINT('Origin',(1.11022302462516E-15,3.05,-16.8941925465839)) ;
#8702=CARTESIAN_POINT('',(11.7,3.05,-28.65)) ;
#8703=CARTESIAN_POINT('Origin',(1.11022302462516E-15,3.05,-16.8941925465839)) ;
#8704=CARTESIAN_POINT('Ctrl Pts',(11.5234344017195,3.3,-28.4730122076873)) ;
#8705=CARTESIAN_POINT('Ctrl Pts',(11.5248174913711,3.3,-28.4743986171276)) ;
#8706=CARTESIAN_POINT('Ctrl Pts',(11.5262005335001,3.29997698962269,-28.4757849786486)) ;
#8707=CARTESIAN_POINT('Ctrl Pts',(11.5499521209721,3.29918654602495,-28.4995935660222)) ;
#8708=CARTESIAN_POINT('Ctrl Pts',(11.5720185826081,3.29242837601996,-28.5217129029717)) ;
#8709=CARTESIAN_POINT('Ctrl Pts',(11.6137589203932,3.26726387117987,-28.5635531294919)) ;
#8710=CARTESIAN_POINT('Ctrl Pts',(11.6329511205595,3.24878239907886,-28.582791187992)) ;
#8711=CARTESIAN_POINT('Ctrl Pts',(11.6652519474717,3.20244341327706,-28.6151691262907)) ;
#8712=CARTESIAN_POINT('Ctrl Pts',(11.6780517643177,3.17502893211499,-28.62799946099)) ;
#8713=CARTESIAN_POINT('Ctrl Pts',(11.6955092411613,3.11479613681801,-28.6454985466269)) ;
#8714=CARTESIAN_POINT('Ctrl Pts',(11.7,3.08255368454763,-28.65)) ;
#8715=CARTESIAN_POINT('Ctrl Pts',(11.7,3.05,-28.65)) ;
#8716=CARTESIAN_POINT('Origin',(21.8132129304798,3.05,-18.1832336789269)) ;
#8717=CARTESIAN_POINT('',(21.9899896257764,3.05,-18.3600103742236)) ;
#8718=CARTESIAN_POINT('Origin',(-24.5,3.05,-7.145)) ;
#8719=CARTESIAN_POINT('',(-24.75,3.05,33.25)) ;
#8720=CARTESIAN_POINT('',(-24.75,3.05,-7.145)) ;
#8721=CARTESIAN_POINT('Origin',(-24.5,3.05,33.25)) ;
#8722=CARTESIAN_POINT('Origin',(24.5,3.05,16.63)) ;
#8723=CARTESIAN_POINT('',(24.75,3.05,33.25)) ;
#8724=CARTESIAN_POINT('Origin',(24.5,3.05,33.25)) ;
#8725=CARTESIAN_POINT('',(24.75,3.05,16.63)) ;
#8726=CARTESIAN_POINT('Origin',(-12.2500207484472,3.05,33.25)) ;
#8727=CARTESIAN_POINT('',(-24.5,3.05,33.5)) ;
#8728=CARTESIAN_POINT('Origin',(-24.5,3.05,33.25)) ;
#8729=CARTESIAN_POINT('',(-10.77,3.05,33.5)) ;
#8730=CARTESIAN_POINT('',(-12.2500207484472,3.05,33.5)) ;
#8731=CARTESIAN_POINT('Origin',(-10.77,3.05,33.25)) ;
#8732=CARTESIAN_POINT('Origin',(-10.77,4.57,33.25)) ;
#8733=CARTESIAN_POINT('',(-9.25,4.57,33.5)) ;
#8734=CARTESIAN_POINT('',(-9.5,4.57,33.25)) ;
#8735=CARTESIAN_POINT('Origin',(-9.25,4.57,33.25)) ;
#8736=CARTESIAN_POINT('Origin',(-10.77,4.57,33.25)) ;
#8737=CARTESIAN_POINT('Origin',(-10.77,4.57,33.5)) ;
#8738=CARTESIAN_POINT('Origin',(-9.25,8.6875,33.25)) ;
#8739=CARTESIAN_POINT('',(-9.25,24.6003192917499,33.5)) ;
#8740=CARTESIAN_POINT('',(-9.5,24.6003192917499,33.25)) ;
#8741=CARTESIAN_POINT('Origin',(-9.25,24.6003192917499,33.25)) ;
#8742=CARTESIAN_POINT('',(-9.5,8.6875,33.25)) ;
#8743=CARTESIAN_POINT('',(-9.25,8.6875,33.5)) ;
#8744=CARTESIAN_POINT('Ctrl Pts',(-9.25,24.6003192917499,33.5)) ;
#8745=CARTESIAN_POINT('Ctrl Pts',(-9.25,25.370369005669,33.5)) ;
#8746=CARTESIAN_POINT('Ctrl Pts',(-8.81719996776914,27.1694431484448,33.5)) ;
#8747=CARTESIAN_POINT('Ctrl Pts',(-7.54929504861548,28.2003141923527,33.5)) ;
#8748=CARTESIAN_POINT('Ctrl Pts',(-6.76795090667124,28.3557987366091,33.5)) ;
#8749=CARTESIAN_POINT('Ctrl Pts',(-9.31544984694979,24.6003192917499,33.5)) ;
#8750=CARTESIAN_POINT('Ctrl Pts',(-9.31001237129096,25.3805985297588,33.4998240176448)) ;
#8751=CARTESIAN_POINT('Ctrl Pts',(-8.85942127194599,27.1975612821968,33.4998356946794)) ;
#8752=CARTESIAN_POINT('Ctrl Pts',(-7.56933624934574,28.2354900210942,33.5000078650668)) ;
#8753=CARTESIAN_POINT('Ctrl Pts',(-6.77517359820447,28.3920943552222,33.5)) ;
#8754=CARTESIAN_POINT('Ctrl Pts',(-9.44567143792189,24.6003192917499,33.4456714379219)) ;
#8755=CARTESIAN_POINT('Ctrl Pts',(-9.4298299112322,25.4008861366219,33.4551270066274)) ;
#8756=CARTESIAN_POINT('Ctrl Pts',(-8.94398652948135,27.2537008535442,33.4736901555626)) ;
#8757=CARTESIAN_POINT('Ctrl Pts',(-7.60938939076493,28.3057987139221,33.4819757476224)) ;
#8758=CARTESIAN_POINT('Ctrl Pts',(-6.789611851291,28.464649762726,33.483268532741)) ;
#8759=CARTESIAN_POINT('Ctrl Pts',(-9.5,24.6003192917499,33.3154498469498)) ;
#8760=CARTESIAN_POINT('Ctrl Pts',(-9.49134428057035,25.4094606950313,33.342417324315)) ;
#8761=CARTESIAN_POINT('Ctrl Pts',(-9.00760901658298,27.2899950446831,33.4011943379152)) ;
#8762=CARTESIAN_POINT('Ctrl Pts',(-7.64149663567344,28.3614500536775,33.4317712233585)) ;
#8763=CARTESIAN_POINT('Ctrl Pts',(-6.80125367349474,28.5231524880223,33.4364220663262)) ;
#8764=CARTESIAN_POINT('Ctrl Pts',(-9.5,24.6003192917499,33.25)) ;
#8765=CARTESIAN_POINT('Ctrl Pts',(-9.5,25.4093792116268,33.2823374075703)) ;
#8766=CARTESIAN_POINT('Ctrl Pts',(-9.03020851202291,27.2995932530022,33.3578875866726)) ;
#8767=CARTESIAN_POINT('Ctrl Pts',(-7.65393565106124,28.3826875378412,33.4011779048128)) ;
#8768=CARTESIAN_POINT('Ctrl Pts',(-6.80580995852349,28.5460488256182,33.407707310626)) ;
#8769=CARTESIAN_POINT('',(-7.77490213744258,27.9,33.5)) ;
#8770=CARTESIAN_POINT('',(-6.80580995852373,28.5460488256181,33.407707310626)) ;
#8771=CARTESIAN_POINT('Ctrl Pts',(-7.77490213744258,27.9,33.5)) ;
#8772=CARTESIAN_POINT('Ctrl Pts',(-7.78114603380676,27.9,33.5)) ;
#8773=CARTESIAN_POINT('Ctrl Pts',(-7.78788956564949,27.9005807447427,33.4999170364653)) ;
#8774=CARTESIAN_POINT('Ctrl Pts',(-7.79738323625925,27.9036098316155,33.4994843097692)) ;
#8775=CARTESIAN_POINT('Ctrl Pts',(-7.80075984355882,27.9052369392644,33.4992518658196)) ;
#8776=CARTESIAN_POINT('Ctrl Pts',(-7.8058478238372,27.9094255221287,33.498653496839)) ;
#8777=CARTESIAN_POINT('Ctrl Pts',(-7.80764775880098,27.9116123995803,33.4983410857742)) ;
#8778=CARTESIAN_POINT('Ctrl Pts',(-7.81039359400954,27.9168212609468,33.4975969627219)) ;
#8779=CARTESIAN_POINT('Ctrl Pts',(-7.81121069749947,27.9197085232834,33.4971844966738)) ;
#8780=CARTESIAN_POINT('Ctrl Pts',(-7.81218916899328,27.927178867045,33.4961173047079)) ;
#8781=CARTESIAN_POINT('Ctrl Pts',(-7.81180402710554,27.9318932870624,33.4954438161339)) ;
#8782=CARTESIAN_POINT('Ctrl Pts',(-7.80918949730732,27.9458600663565,33.4934485619491)) ;
#8783=CARTESIAN_POINT('Ctrl Pts',(-7.80504750550433,27.9558650275853,33.4920192817735)) ;
#8784=CARTESIAN_POINT('Ctrl Pts',(-7.78977167890809,27.9863923872478,33.4876582303932)) ;
#8785=CARTESIAN_POINT('Ctrl Pts',(-7.77102732566492,28.0128597160257,33.483877183425)) ;
#8786=CARTESIAN_POINT('Ctrl Pts',(-7.68861250822215,28.1074719134625,33.4703611552197)) ;
#8787=CARTESIAN_POINT('Ctrl Pts',(-7.59512622632696,28.1900482534497,33.4585645351902)) ;
#8788=CARTESIAN_POINT('Ctrl Pts',(-7.29573476020478,28.3831508397044,33.4309784514395)) ;
#8789=CARTESIAN_POINT('Ctrl Pts',(-7.07088849616787,28.486213422642,33.4162552253368)) ;
#8790=CARTESIAN_POINT('Ctrl Pts',(-6.80580995852349,28.5460488256182,33.407707310626)) ;
#8791=CARTESIAN_POINT('Origin',(-6.325,24.6003192917499,33.25)) ;
#8792=CARTESIAN_POINT('Origin',(-6.325,24.6003192917499,33.5)) ;
#8793=CARTESIAN_POINT('Origin',(-24.5,3.05,33.25)) ;
#8794=CARTESIAN_POINT('Origin',(-24.5,3.05,33.25)) ;
#8795=CARTESIAN_POINT('Origin',(24.5,3.05,33.25)) ;
#8796=CARTESIAN_POINT('Origin',(24.5,3.05,33.25)) ;
#8797=CARTESIAN_POINT('Origin',(9.5,17.375,2.475)) ;
#8798=CARTESIAN_POINT('',(9.5,4.57,-28.55)) ;
#8799=CARTESIAN_POINT('',(9.5,4.57,1.2425)) ;
#8800=CARTESIAN_POINT('',(9.5,12.6602026834209,-28.55)) ;
#8801=CARTESIAN_POINT('',(9.5,3.,-28.55)) ;
#8802=CARTESIAN_POINT('',(9.5,28.157290298199,23.106958715927)) ;
#8803=CARTESIAN_POINT('',(9.5,17.5986951224045,-12.0883585367213)) ;
#8804=CARTESIAN_POINT('',(9.5,28.5749851188244,25.8674171460039)) ;
#8805=CARTESIAN_POINT('Origin',(9.5,18.3909804312853,25.996564592546)) ;
#8806=CARTESIAN_POINT('',(9.5,28.575,14.1625)) ;
#8807=CARTESIAN_POINT('Origin',(10.77,4.57,1.2425)) ;
#8808=CARTESIAN_POINT('Origin',(10.77,4.57,-29.82)) ;
#8809=CARTESIAN_POINT('Origin',(-4.14968943118765E-5,3.3,0.0099999999999989)) ;
#8810=CARTESIAN_POINT('',(-4.75002074844716,3.3,-29.82)) ;
#8811=CARTESIAN_POINT('Origin',(-4.75002074844716,4.57,-29.82)) ;
#8812=CARTESIAN_POINT('',(-9.5,4.57,-28.55)) ;
#8813=CARTESIAN_POINT('Origin',(-10.77,4.57,-29.82)) ;
#8814=CARTESIAN_POINT('',(-4.75002074844716,4.57,-28.55)) ;
#8815=CARTESIAN_POINT('Origin',(-10.77,4.57,1.2425)) ;
#8816=CARTESIAN_POINT('',(-9.5,4.57,1.2425)) ;
#8817=CARTESIAN_POINT('Origin',(-9.5,17.375,2.475)) ;
#8818=CARTESIAN_POINT('',(-9.5,28.575,28.455147082111)) ;
#8819=CARTESIAN_POINT('',(-9.5,33.0419144924728,23.0664883292866)) ;
#8820=CARTESIAN_POINT('',(-9.5,28.575,25.8674157457972)) ;
#8821=CARTESIAN_POINT('',(-9.5,28.575,14.1625)) ;
#8822=CARTESIAN_POINT('',(-9.5,28.1572902981989,23.1069587159267)) ;
#8823=CARTESIAN_POINT('Origin',(-9.5,18.3909804312853,25.996564592546)) ;
#8824=CARTESIAN_POINT('',(-9.5,12.6602026834209,-28.55)) ;
#8825=CARTESIAN_POINT('',(-9.5,17.5986951224045,-12.0883585367213)) ;
#8826=CARTESIAN_POINT('',(-9.5,3.,-28.55)) ;
#8827=CARTESIAN_POINT('Origin',(-6.325,33.0419144924728,23.0664883292866)) ;
#8828=CARTESIAN_POINT('Origin',(-6.325,28.575,28.455147082111)) ;
#8829=CARTESIAN_POINT('Origin',(-6.325,23.9220039727312,34.0682851467527)) ;
#8830=CARTESIAN_POINT('Origin',(6.325,18.3909804312853,25.996564592546)) ;
#8831=CARTESIAN_POINT('',(6.325,31.2,22.2)) ;
#8832=CARTESIAN_POINT('',(6.325,31.75,25.85)) ;
#8833=CARTESIAN_POINT('Origin',(6.325,18.3909804312853,25.996564592546)) ;
#8834=CARTESIAN_POINT('Ctrl Pts',(6.325,31.75,25.85)) ;
#8835=CARTESIAN_POINT('Ctrl Pts',(6.43046220354674,31.74999470036,25.8495169502164)) ;
#8836=CARTESIAN_POINT('Ctrl Pts',(6.53592423385766,31.7447307283387,25.8490915953681)) ;
#8837=CARTESIAN_POINT('Ctrl Pts',(6.64086325133653,31.7342341731504,25.8487253551069)) ;
#8838=CARTESIAN_POINT('Ctrl Pts',(6.74579915993031,31.7237379289293,25.8483591256958)) ;
#8839=CARTESIAN_POINT('Ctrl Pts',(6.85021174198924,31.7080094463137,25.8480520088604)) ;
#8840=CARTESIAN_POINT('Ctrl Pts',(6.95358339129659,31.6871266888496,25.847804826769)) ;
#8841=CARTESIAN_POINT('Ctrl Pts',(7.05695217787227,31.666244509704,25.847557651523)) ;
#8842=CARTESIAN_POINT('Ctrl Pts',(7.15927974986701,31.6402084100166,25.847370408779)) ;
#8843=CARTESIAN_POINT('Ctrl Pts',(7.260058865173,31.6091474441695,25.8472433040211)) ;
#8844=CARTESIAN_POINT('Ctrl Pts',(7.3608353843029,31.5780872784856,25.8471162025376)) ;
#8845=CARTESIAN_POINT('Ctrl Pts',(7.4600631956079,31.5420026077587,25.847049236588)) ;
#8846=CARTESIAN_POINT('Ctrl Pts',(7.55725044792966,31.5010722880811,25.8470419821051)) ;
#8847=CARTESIAN_POINT('Ctrl Pts',(7.6544353845022,31.460142943679,25.8470347277951)) ;
#8848=CARTESIAN_POINT('Ctrl Pts',(7.74957954026074,31.4143683158502,25.8470871823076)) ;
#8849=CARTESIAN_POINT('Ctrl Pts',(7.84221132830012,31.363975280532,25.847198285725)) ;
#8850=CARTESIAN_POINT('Ctrl Pts',(7.934841088328,31.3135833484815,25.8473093867099)) ;
#8851=CARTESIAN_POINT('Ctrl Pts',(8.0249582865672,31.2585733768047,25.8474791337795)) ;
#8852=CARTESIAN_POINT('Ctrl Pts',(8.1121162720151,31.199218004425,25.8477058315995)) ;
#8853=CARTESIAN_POINT('Ctrl Pts',(8.19927251801032,31.1398638166283,25.8479325248951)) ;
#8854=CARTESIAN_POINT('Ctrl Pts',(8.28346938325736,31.0761645966036,25.8482161659582)) ;
#8855=CARTESIAN_POINT('Ctrl Pts',(8.36428957653771,31.0084360368315,25.8485544313)) ;
#8856=CARTESIAN_POINT('Ctrl Pts',(8.44510831342536,30.9407086975387,25.8488926905462)) ;
#8857=CARTESIAN_POINT('Ctrl Pts',(8.52255023480056,30.8689523861978,25.8492855709361)) ;
#8858=CARTESIAN_POINT('Ctrl Pts',(8.59623154168566,30.7935227137269,25.8497301349389)) ;
#8859=CARTESIAN_POINT('Ctrl Pts',(8.66992458575925,30.7180810255587,25.8501747697592)) ;
#8860=CARTESIAN_POINT('Ctrl Pts',(8.73985557411532,30.6389650526736,25.8506711030591)) ;
#8861=CARTESIAN_POINT('Ctrl Pts',(8.80567782139028,30.5565670039655,25.8512156022673)) ;
#8862=CARTESIAN_POINT('Ctrl Pts',(8.87149635540453,30.4741736036164,25.8517600707585)) ;
#8863=CARTESIAN_POINT('Ctrl Pts',(8.9332063960891,30.388498768684,25.8523526976616)) ;
#8864=CARTESIAN_POINT('Ctrl Pts',(8.99050204818587,30.2999671749436,25.8529893849969)) ;
#8865=CARTESIAN_POINT('Ctrl Pts',(9.04779491311263,30.2114398878581,25.8536260413604)) ;
#8866=CARTESIAN_POINT('Ctrl Pts',(9.10067363112342,30.1200564108484,25.8543067513843)) ;
#8867=CARTESIAN_POINT('Ctrl Pts',(9.1488761090875,30.0262696721175,25.8550268858408)) ;
#8868=CARTESIAN_POINT('Ctrl Pts',(9.19707661659256,29.9324867672751,25.8557469908591)) ;
#8869=CARTESIAN_POINT('Ctrl Pts',(9.2406011084124,29.8363011052836,25.8565065141989)) ;
#8870=CARTESIAN_POINT('Ctrl Pts',(9.27923387320771,29.7381893761549,25.8573003357022)) ;
#8871=CARTESIAN_POINT('Ctrl Pts',(9.317871729721,29.6400647161046,25.8580942618295)) ;
#8872=CARTESIAN_POINT('Ctrl Pts',(9.35161644172219,29.5400138030315,25.8589224919069)) ;
#8873=CARTESIAN_POINT('Ctrl Pts',(9.38030072332849,29.4385326126193,25.8597794581924)) ;
#8874=CARTESIAN_POINT('Ctrl Pts',(9.40898209837118,29.3370617052442,25.860636337642)) ;
#8875=CARTESIAN_POINT('Ctrl Pts',(9.43260397516068,29.234161143853,25.8615219438564)) ;
#8876=CARTESIAN_POINT('Ctrl Pts',(9.4510492744072,29.1303409262827,25.8624303169636)) ;
#8877=CARTESIAN_POINT('Ctrl Pts',(9.4694959506141,29.0265129584274,25.8633387578817)) ;
#8878=CARTESIAN_POINT('Ctrl Pts',(9.48276521515409,28.921765537959,25.8642699651669)) ;
#8879=CARTESIAN_POINT('Ctrl Pts',(9.49079129054069,28.8166178923319,25.8652176403169)) ;
#8880=CARTESIAN_POINT('Ctrl Pts',(9.49692746081675,28.7362294301487,25.8659421657925)) ;
#8881=CARTESIAN_POINT('Ctrl Pts',(9.5,28.6556072605121,25.8666763094571)) ;
#8882=CARTESIAN_POINT('Ctrl Pts',(9.5,28.5749851188244,25.8674171460039)) ;
#8883=CARTESIAN_POINT('Ctrl Pts',(9.5,28.157290298199,23.106958715927)) ;
#8884=CARTESIAN_POINT('Ctrl Pts',(9.5,28.1804450776003,23.1000600670451)) ;
#8885=CARTESIAN_POINT('Ctrl Pts',(9.49972422059564,28.203599079594,23.0931615647751)) ;
#8886=CARTESIAN_POINT('Ctrl Pts',(9.4985130472546,28.2544365009203,23.0780148814088)) ;
#8887=CARTESIAN_POINT('Ctrl Pts',(9.49745895112732,28.2821152676473,23.0697680502854)) ;
#8888=CARTESIAN_POINT('Ctrl Pts',(9.49333672763788,28.3608494434134,23.0463090288973)) ;
#8889=CARTESIAN_POINT('Ctrl Pts',(9.48931972873393,28.4118497186112,23.031112980272)) ;
#8890=CARTESIAN_POINT('Ctrl Pts',(9.47326463912736,28.5643586303592,22.985670233064)) ;
#8891=CARTESIAN_POINT('Ctrl Pts',(9.45723262679727,28.6654075247228,22.9555593489331)) ;
#8892=CARTESIAN_POINT('Ctrl Pts',(9.39330812722704,28.965714961593,22.8660684272176)) ;
#8893=CARTESIAN_POINT('Ctrl Pts',(9.32974954840376,29.1613140148577,22.8077745275644)) ;
#8894=CARTESIAN_POINT('Ctrl Pts',(9.08425034832404,29.7138633169295,22.64308623758)) ;
#8895=CARTESIAN_POINT('Ctrl Pts',(8.84953554453401,30.0445944579936,22.5444934762977)) ;
#8896=CARTESIAN_POINT('Ctrl Pts',(8.26103034811584,30.6012160783936,22.3785462415353)) ;
#8897=CARTESIAN_POINT('Ctrl Pts',(7.91286656009489,30.8217851943026,22.3127786094015)) ;
#8898=CARTESIAN_POINT('Ctrl Pts',(7.14791041241991,31.1226151396577,22.2230766109168)) ;
#8899=CARTESIAN_POINT('Ctrl Pts',(6.73843153640591,31.2000000000001,22.2000000000002)) ;
#8900=CARTESIAN_POINT('Ctrl Pts',(6.325,31.2000000000001,22.2000000000003)) ;
#8901=CARTESIAN_POINT('Origin',(6.325,28.575,14.1625)) ;
#8902=CARTESIAN_POINT('',(6.325,31.75,14.1625)) ;
#8903=CARTESIAN_POINT('Origin',(6.325,17.5986951224045,-12.0883585367213)) ;
#8904=CARTESIAN_POINT('',(9.36972204690191,13.6,-28.55)) ;
#8905=CARTESIAN_POINT('Origin',(6.325,12.6602026834209,-28.55)) ;
#8906=CARTESIAN_POINT('',(6.325,16.65,-26.3)) ;
#8907=CARTESIAN_POINT('Ctrl Pts',(9.36972204690191,13.6,-28.55)) ;
#8908=CARTESIAN_POINT('Ctrl Pts',(9.33150428640196,13.7352848730332,-28.5489172081766)) ;
#8909=CARTESIAN_POINT('Ctrl Pts',(9.28537554981067,13.8692960232194,-28.5392936237713)) ;
#8910=CARTESIAN_POINT('Ctrl Pts',(9.06189751586222,14.4233292907506,-28.4655098589506)) ;
#8911=CARTESIAN_POINT('Ctrl Pts',(8.81830342317927,14.8140076105995,-28.324179740912)) ;
#8912=CARTESIAN_POINT('Ctrl Pts',(8.20202480438423,15.5807535317409,-27.9023312808353)) ;
#8913=CARTESIAN_POINT('Ctrl Pts',(7.77008447929203,15.9418765716257,-27.5554690453292)) ;
#8914=CARTESIAN_POINT('Ctrl Pts',(7.18160415304357,16.3103729693986,-27.046927007198)) ;
#8915=CARTESIAN_POINT('Ctrl Pts',(6.98513622894908,16.4114752355335,-26.8706894533264)) ;
#8916=CARTESIAN_POINT('Ctrl Pts',(6.7262959895539,16.524579645383,-26.6336670195021)) ;
#8917=CARTESIAN_POINT('Ctrl Pts',(6.64224012239147,16.5576770884375,-26.5557152165318)) ;
#8918=CARTESIAN_POINT('Ctrl Pts',(6.52704506600961,16.5986811618034,-26.4494819237855)) ;
#8919=CARTESIAN_POINT('Ctrl Pts',(6.48975900833928,16.611175247101,-26.4152486293163)) ;
#8920=CARTESIAN_POINT('Ctrl Pts',(6.43498907397076,16.6280885098712,-26.3665958960957)) ;
#8921=CARTESIAN_POINT('Ctrl Pts',(6.41711081442205,16.6333341653242,-26.3511046831613)) ;
#8922=CARTESIAN_POINT('Ctrl Pts',(6.38827974448016,16.6407770204755,-26.3285991010218)) ;
#8923=CARTESIAN_POINT('Ctrl Pts',(6.37860103000991,16.6431409047043,-26.3213573070103)) ;
#8924=CARTESIAN_POINT('Ctrl Pts',(6.36186612440196,16.6464275938578,-26.3111801406621)) ;
#8925=CARTESIAN_POINT('Ctrl Pts',(6.35597562166154,16.6474585886992,-26.3079691091064)) ;
#8926=CARTESIAN_POINT('Ctrl Pts',(6.34245949856352,16.6492439669154,-26.3023795561698)) ;
#8927=CARTESIAN_POINT('Ctrl Pts',(6.33483452413194,16.65,-26.2999999999999)) ;
#8928=CARTESIAN_POINT('Ctrl Pts',(6.325,16.65,-26.2999999999999)) ;
#8929=CARTESIAN_POINT('',(6.325,20.6397935779816,-13.0006880733945)) ;
#8930=CARTESIAN_POINT('Origin',(-9.5,28.6,33.4)) ;
#8931=CARTESIAN_POINT('',(-9.5,27.9,33.5)) ;
#8932=CARTESIAN_POINT('Origin',(-9.5,31.75,25.85)) ;
#8933=CARTESIAN_POINT('',(-6.325,31.75,25.85)) ;
#8934=CARTESIAN_POINT('',(-9.5,31.75,25.85)) ;
#8935=CARTESIAN_POINT('',(-6.325,31.75,14.1625)) ;
#8936=CARTESIAN_POINT('Origin',(-9.5,18.3909804312853,25.996564592546)) ;
#8937=CARTESIAN_POINT('',(-6.325,31.2,22.2)) ;
#8938=CARTESIAN_POINT('',(-9.5,31.2,22.2)) ;
#8939=CARTESIAN_POINT('Origin',(-6.325,18.3909804312853,25.996564592546)) ;
#8940=CARTESIAN_POINT('Origin',(-9.5,16.65,-26.3)) ;
#8941=CARTESIAN_POINT('',(-6.325,16.65,-26.3)) ;
#8942=CARTESIAN_POINT('',(-9.5,16.65,-26.3)) ;
#8943=CARTESIAN_POINT('',(-6.325,20.6397935779816,-13.0006880733945)) ;
#8944=CARTESIAN_POINT('Origin',(-9.5,13.5741698750304,-25.3227636083745)) ;
#8945=CARTESIAN_POINT('',(-9.36972204690191,13.6,-28.55)) ;
#8946=CARTESIAN_POINT('',(-9.5,13.6,-28.55)) ;
#8947=CARTESIAN_POINT('Ctrl Pts',(-6.325,16.65,-26.2999999999999)) ;
#8948=CARTESIAN_POINT('Ctrl Pts',(-6.33483452413193,16.65,-26.2999999999999)) ;
#8949=CARTESIAN_POINT('Ctrl Pts',(-6.34245949856349,16.6492439669154,-26.3023795561699)) ;
#8950=CARTESIAN_POINT('Ctrl Pts',(-6.35597562166151,16.6474585886992,-26.3079691091065)) ;
#8951=CARTESIAN_POINT('Ctrl Pts',(-6.36186612440198,16.6464275938579,-26.311180140662)) ;
#8952=CARTESIAN_POINT('Ctrl Pts',(-6.37860103000995,16.6431409047044,-26.3213573070102)) ;
#8953=CARTESIAN_POINT('Ctrl Pts',(-6.38827974448013,16.6407770204755,-26.3285991010219)) ;
#8954=CARTESIAN_POINT('Ctrl Pts',(-6.41711081442201,16.6333341653242,-26.3511046831614)) ;
#8955=CARTESIAN_POINT('Ctrl Pts',(-6.43498907397077,16.6280885098712,-26.3665958960957)) ;
#8956=CARTESIAN_POINT('Ctrl Pts',(-6.4897590083393,16.611175247101,-26.4152486293163)) ;
#8957=CARTESIAN_POINT('Ctrl Pts',(-6.52704506600962,16.5986811618034,-26.4494819237855)) ;
#8958=CARTESIAN_POINT('Ctrl Pts',(-6.64224012239148,16.5576770884375,-26.5557152165318)) ;
#8959=CARTESIAN_POINT('Ctrl Pts',(-6.72629598955389,16.524579645383,-26.6336670195021)) ;
#8960=CARTESIAN_POINT('Ctrl Pts',(-6.98513622894906,16.4114752355335,-26.8706894533264)) ;
#8961=CARTESIAN_POINT('Ctrl Pts',(-7.18160415304355,16.3103729693986,-27.0469270071979)) ;
#8962=CARTESIAN_POINT('Ctrl Pts',(-7.770084479292,15.9418765716257,-27.5554690453291)) ;
#8963=CARTESIAN_POINT('Ctrl Pts',(-8.2020248043842,15.5807535317409,-27.9023312808353)) ;
#8964=CARTESIAN_POINT('Ctrl Pts',(-8.81830342317925,14.8140076105995,-28.324179740912)) ;
#8965=CARTESIAN_POINT('Ctrl Pts',(-9.06189751586222,14.4233292907506,-28.4655098589506)) ;
#8966=CARTESIAN_POINT('Ctrl Pts',(-9.28537554981067,13.8692960232194,-28.5392936237713)) ;
#8967=CARTESIAN_POINT('Ctrl Pts',(-9.33150428640196,13.7352848730332,-28.5489172081766)) ;
#8968=CARTESIAN_POINT('Ctrl Pts',(-9.36972204690191,13.6,-28.55)) ;
#8969=CARTESIAN_POINT('Origin',(-6.325,17.5986951224045,-12.0883585367213)) ;
#8970=CARTESIAN_POINT('Origin',(-6.325,12.6602026834209,-28.55)) ;
#8971=CARTESIAN_POINT('Ctrl Pts',(-9.5,28.1572902981989,23.1069587159267)) ;
#8972=CARTESIAN_POINT('Ctrl Pts',(-9.5,28.1804450776062,23.100060067043)) ;
#8973=CARTESIAN_POINT('Ctrl Pts',(-9.49972422059572,28.203599079597,23.0931615647918)) ;
#8974=CARTESIAN_POINT('Ctrl Pts',(-9.49851304725432,28.2544365009326,23.0780148814129)) ;
#8975=CARTESIAN_POINT('Ctrl Pts',(-9.49745895112744,28.282115267648,23.0697680502973)) ;
#8976=CARTESIAN_POINT('Ctrl Pts',(-9.49333672763735,28.3608494434262,23.0463090289002)) ;
#8977=CARTESIAN_POINT('Ctrl Pts',(-9.48931972873404,28.4118497186098,23.0311129802741)) ;
#8978=CARTESIAN_POINT('Ctrl Pts',(-9.47326463912794,28.5643586303556,22.9856702330659)) ;
#8979=CARTESIAN_POINT('Ctrl Pts',(-9.45723262679847,28.6654075247156,22.9555593489356)) ;
#8980=CARTESIAN_POINT('Ctrl Pts',(-9.39330812723007,28.9657149615822,22.8660684272212)) ;
#8981=CARTESIAN_POINT('Ctrl Pts',(-9.32974954840784,29.1613140148454,22.8077745275693)) ;
#8982=CARTESIAN_POINT('Ctrl Pts',(-9.08425034833606,29.7138633169093,22.6430862375867)) ;
#8983=CARTESIAN_POINT('Ctrl Pts',(-8.84953554453545,30.0445944579962,22.544493476295)) ;
#8984=CARTESIAN_POINT('Ctrl Pts',(-8.26103034809262,30.6012160784109,22.378546241529)) ;
#8985=CARTESIAN_POINT('Ctrl Pts',(-7.91286656008235,30.8217851943076,22.3127786094003)) ;
#8986=CARTESIAN_POINT('Ctrl Pts',(-7.14791041242474,31.1226151396559,22.2230766109175)) ;
#8987=CARTESIAN_POINT('Ctrl Pts',(-6.73843153640695,31.2000000000001,22.2000000000002)) ;
#8988=CARTESIAN_POINT('Ctrl Pts',(-6.325,31.2000000000001,22.2000000000002)) ;
#8989=CARTESIAN_POINT('Origin',(-6.325,28.575,14.1625)) ;
#8990=CARTESIAN_POINT('Ctrl Pts',(-6.325,31.75,25.85)) ;
#8991=CARTESIAN_POINT('Ctrl Pts',(-6.43046239133936,31.75,25.8503682782621)) ;
#8992=CARTESIAN_POINT('Ctrl Pts',(-6.53592460944136,31.7447410186195,25.8507365565242)) ;
#8993=CARTESIAN_POINT('Ctrl Pts',(-6.64086381191953,31.7342491279289,25.8511048347863)) ;
#8994=CARTESIAN_POINT('Ctrl Pts',(-6.74579990719284,31.7237575478987,25.8514731021438)) ;
#8995=CARTESIAN_POINT('Ctrl Pts',(-6.8502126731198,31.7080334031633,25.8518413695013)) ;
#8996=CARTESIAN_POINT('Ctrl Pts',(-6.95358450071494,31.6871546435646,25.8522096368589)) ;
#8997=CARTESIAN_POINT('Ctrl Pts',(-7.05695346822128,31.6662764616389,25.8525778940272)) ;
#8998=CARTESIAN_POINT('Ctrl Pts',(-7.15928121551033,31.6402440188948,25.8529461511955)) ;
#8999=CARTESIAN_POINT('Ctrl Pts',(-7.26006049775935,31.6091863597232,25.8533144083638)) ;
#9000=CARTESIAN_POINT('Ctrl Pts',(-7.3608371872827,31.5781294995648,25.8536826560581)) ;
#9001=CARTESIAN_POINT('Ctrl Pts',(-7.46006516052103,31.542047783755,25.8540509037523)) ;
#9002=CARTESIAN_POINT('Ctrl Pts',(-7.55725256368973,31.5011200623488,25.8544191514466)) ;
#9003=CARTESIAN_POINT('Ctrl Pts',(-7.6544376551641,31.4601933144471,25.8547873903817)) ;
#9004=CARTESIAN_POINT('Ctrl Pts',(-7.74958195456512,31.4144209260739,25.8551556293169)) ;
#9005=CARTESIAN_POINT('Ctrl Pts',(-7.84221387248779,31.364029771288,25.855523868252)) ;
#9006=CARTESIAN_POINT('Ctrl Pts',(-7.93484376682315,31.3136397173203,25.8558920991428)) ;
#9007=CARTESIAN_POINT('Ctrl Pts',(-8.02496108536813,31.2586312643688,25.8562603300335)) ;
#9008=CARTESIAN_POINT('Ctrl Pts',(-8.11211917478788,31.1992770538008,25.8566285609243)) ;
#9009=CARTESIAN_POINT('Ctrl Pts',(-8.19927552929977,31.1399240246962,25.8569967844854)) ;
#9010=CARTESIAN_POINT('Ctrl Pts',(-8.28347248641858,31.0762256060054,25.8573650080464)) ;
#9011=CARTESIAN_POINT('Ctrl Pts',(-8.36429275280517,31.0084974970927,25.8577332316074)) ;
#9012=CARTESIAN_POINT('Ctrl Pts',(-8.44511156722147,30.9407706049441,25.8581014485532)) ;
#9013=CARTESIAN_POINT('Ctrl Pts',(-8.52255354698811,30.8690143898423,25.8584696654989)) ;
#9014=CARTESIAN_POINT('Ctrl Pts',(-8.59623489126445,30.7935844740967,25.8588378824447)) ;
#9015=CARTESIAN_POINT('Ctrl Pts',(-8.66992797872015,30.718142536488,25.8592061580761)) ;
#9016=CARTESIAN_POINT('Ctrl Pts',(-8.73985898883772,30.6390259739448,25.8595744337075)) ;
#9017=CARTESIAN_POINT('Ctrl Pts',(-8.80568123466801,30.5566270113132,25.8599427093388)) ;
#9018=CARTESIAN_POINT('Ctrl Pts',(-8.87149977051629,30.4742326929879,25.8603109642129)) ;
#9019=CARTESIAN_POINT('Ctrl Pts',(-8.93320978941985,30.3885566155287,25.8606792190869)) ;
#9020=CARTESIAN_POINT('Ctrl Pts',(-8.9905053948943,30.3000234751415,25.861047473961)) ;
#9021=CARTESIAN_POINT('Ctrl Pts',(-9.04779821585521,30.2114946373833,25.8614157109381)) ;
#9022=CARTESIAN_POINT('Ctrl Pts',(-9.10067686465044,30.1201093053544,25.8617839479153)) ;
#9023=CARTESIAN_POINT('Ctrl Pts',(-9.14887924732489,30.0263204320645,25.8621521848925)) ;
#9024=CARTESIAN_POINT('Ctrl Pts',(-9.19707966154245,29.9325353888623,25.8625204068319)) ;
#9025=CARTESIAN_POINT('Ctrl Pts',(-9.24060403361372,29.836347308807,25.8628886287713)) ;
#9026=CARTESIAN_POINT('Ctrl Pts',(-9.27923665181417,29.7382329109331,25.8632568507106)) ;
#9027=CARTESIAN_POINT('Ctrl Pts',(-9.31787436355134,29.6401055771177,25.8636251211984)) ;
#9028=CARTESIAN_POINT('Ctrl Pts',(-9.35161890345644,29.5400517393644,25.8639933916862)) ;
#9029=CARTESIAN_POINT('Ctrl Pts',(-9.38030298572493,29.4385674064138,25.864361662174)) ;
#9030=CARTESIAN_POINT('Ctrl Pts',(-9.40898416208845,29.3370933545602,25.8647298953533)) ;
#9031=CARTESIAN_POINT('Ctrl Pts',(-9.43260581273696,29.234189430832,25.8650981285326)) ;
#9032=CARTESIAN_POINT('Ctrl Pts',(-9.45105085895399,29.1303656698366,25.8654663617119)) ;
#9033=CARTESIAN_POINT('Ctrl Pts',(-9.46949728240109,29.0265341566673,25.865834622386)) ;
#9034=CARTESIAN_POINT('Ctrl Pts',(-9.4827662671269,28.9217830097633,25.86620288306)) ;
#9035=CARTESIAN_POINT('Ctrl Pts',(-9.49079203672237,28.8166314967574,25.8665711437341)) ;
#9036=CARTESIAN_POINT('Ctrl Pts',(-9.49692771002532,28.7362435260538,25.8668526777551)) ;
#9037=CARTESIAN_POINT('Ctrl Pts',(-9.5,28.6556217856458,25.8671342117762)) ;
#9038=CARTESIAN_POINT('Ctrl Pts',(-9.5,28.575,25.8674157457972)) ;
#9039=CARTESIAN_POINT('Origin',(-6.325,18.3909804312853,25.996564592546)) ;
#9040=CARTESIAN_POINT('Origin',(-9.5,3.,-28.55)) ;
#9041=CARTESIAN_POINT('Origin',(-16.75,0.,12.99)) ;
#9042=CARTESIAN_POINT('',(-16.75,0.,12.99)) ;
#9043=CARTESIAN_POINT('',(-16.75,0.,12.99)) ;
#9044=CARTESIAN_POINT('',(-18.25,0.,12.99)) ;
#9045=CARTESIAN_POINT('Origin',(-16.75,0.,10.325)) ;
#9046=CARTESIAN_POINT('Origin',(-16.75,0.,10.325)) ;
#9047=CARTESIAN_POINT('Origin',(18.25,0.,12.99)) ;
#9048=CARTESIAN_POINT('',(18.25,0.,12.99)) ;
#9049=CARTESIAN_POINT('',(18.25,0.,12.99)) ;
#9050=CARTESIAN_POINT('',(16.75,0.,12.99)) ;
#9051=CARTESIAN_POINT('Origin',(18.25,0.,10.325)) ;
#9052=CARTESIAN_POINT('Origin',(18.25,0.,10.325)) ;
#9053=CARTESIAN_POINT('Origin',(-24.75,0.,-14.3)) ;
#9054=CARTESIAN_POINT('',(-24.75,0.,-14.3)) ;
#9055=CARTESIAN_POINT('',(-24.75,0.,-14.3)) ;
#9056=CARTESIAN_POINT('',(-24.75,0.,33.25)) ;
#9057=CARTESIAN_POINT('',(-24.75,0.,33.25)) ;
#9058=CARTESIAN_POINT('',(-24.75,0.,33.25)) ;
#9059=CARTESIAN_POINT('Origin',(-21.664129241231,0.,-14.3226323462975)) ;
#9060=CARTESIAN_POINT('',(-23.8,0.,-16.55)) ;
#9061=CARTESIAN_POINT('',(-23.8,0.,-16.55)) ;
#9062=CARTESIAN_POINT('Origin',(-21.664129241231,0.,-14.3226323462975)) ;
#9063=CARTESIAN_POINT('Origin',(-11.7,0.,-28.65)) ;
#9064=CARTESIAN_POINT('',(-11.7,0.,-28.65)) ;
#9065=CARTESIAN_POINT('',(-11.7,0.,-28.65)) ;
#9066=CARTESIAN_POINT('',(-23.8,0.,-16.55)) ;
#9067=CARTESIAN_POINT('Origin',(1.11022302462516E-15,0.,-16.8941925465839)) ;
#9068=CARTESIAN_POINT('',(11.7,0.,-28.65)) ;
#9069=CARTESIAN_POINT('',(11.7,0.,-28.65)) ;
#9070=CARTESIAN_POINT('Origin',(1.11022302462516E-15,0.,-16.8941925465839)) ;
#9071=CARTESIAN_POINT('Origin',(23.8,0.,-16.55)) ;
#9072=CARTESIAN_POINT('',(23.8,0.,-16.55)) ;
#9073=CARTESIAN_POINT('',(23.8,0.,-16.55)) ;
#9074=CARTESIAN_POINT('',(11.7,0.,-28.65)) ;
#9075=CARTESIAN_POINT('Origin',(21.4457388066382,0.,-14.2304230516917)) ;
#9076=CARTESIAN_POINT('',(24.75,0.,-14.3)) ;
#9077=CARTESIAN_POINT('',(24.75,0.,-14.3)) ;
#9078=CARTESIAN_POINT('Origin',(21.4457388066382,0.,-14.2304230516917)) ;
#9079=CARTESIAN_POINT('Origin',(24.75,0.,33.25)) ;
#9080=CARTESIAN_POINT('',(24.75,0.,33.25)) ;
#9081=CARTESIAN_POINT('',(24.75,0.,33.25)) ;
#9082=CARTESIAN_POINT('',(24.75,0.,-14.3)) ;
#9083=CARTESIAN_POINT('Origin',(24.5,0.,33.25)) ;
#9084=CARTESIAN_POINT('',(24.5,0.,33.5)) ;
#9085=CARTESIAN_POINT('',(24.5,0.,33.5)) ;
#9086=CARTESIAN_POINT('Origin',(24.5,0.,33.25)) ;
#9087=CARTESIAN_POINT('Origin',(-24.5,0.,33.5)) ;
#9088=CARTESIAN_POINT('',(-24.5,0.,33.5)) ;
#9089=CARTESIAN_POINT('',(-24.5,0.,33.5)) ;
#9090=CARTESIAN_POINT('',(24.5,0.,33.5)) ;
#9091=CARTESIAN_POINT('Origin',(-24.5,0.,33.25)) ;
#9092=CARTESIAN_POINT('Origin',(-24.5,0.,33.25)) ;
#9093=CARTESIAN_POINT('Origin',(-4.14968943118765E-5,0.,0.0099999999999989)) ;
#11364=UNCERTAINTY_MEASURE_WITH_UNIT(LENGTH_MEASURE(0.01),#11397,
'DISTANCE_ACCURACY_VALUE',
'Maximum model space distance between geometric entities at asserted c
onnectivities') ;
#11379=UNCERTAINTY_MEASURE_WITH_UNIT(LENGTH_MEASURE(0.01),#11397,
'DISTANCE_ACCURACY_VALUE',
'Maximum model space distance between geometric entities at asserted c
onnectivities') ;
#11381=(
GEOMETRIC_REPRESENTATION_CONTEXT(3)
GLOBAL_UNCERTAINTY_ASSIGNED_CONTEXT((#11364))
GLOBAL_UNIT_ASSIGNED_CONTEXT((#11397,#11399,#11400))
REPRESENTATION_CONTEXT('','3D')
) ;
#11396=(
GEOMETRIC_REPRESENTATION_CONTEXT(3)
GLOBAL_UNCERTAINTY_ASSIGNED_CONTEXT((#11379))
GLOBAL_UNIT_ASSIGNED_CONTEXT((#11397,#11399,#11400))
REPRESENTATION_CONTEXT('','3D')
) ;
#11397=(
LENGTH_UNIT()
NAMED_UNIT(*)
SI_UNIT(.MILLI.,.METRE.)
) ;
#11399=(
NAMED_UNIT(*)
PLANE_ANGLE_UNIT()
SI_UNIT($,.RADIAN.)
) ;
#11400=(
NAMED_UNIT(*)
SI_UNIT($,.STERADIAN.)
SOLID_ANGLE_UNIT()
) ;
#11402=SHAPE_DEFINITION_REPRESENTATION(#11418,#11455) ;
#11418=PRODUCT_DEFINITION_SHAPE('',$,#11472) ;
#11455=SHAPE_REPRESENTATION('',(#5751),#11381) ;
#11470=PRODUCT_DEFINITION_CONTEXT('part definition',#11520,'design') ;
#11472=PRODUCT_DEFINITION('Latch Housing with Base Plate (cast steel)',
'Latch Housing with Base Plate (cast steel)',#11488,#11470) ;
#11488=PRODUCT_DEFINITION_FORMATION('',$,#11523) ;
#11520=APPLICATION_CONTEXT(
'Core Data for Automotive Mechanical Design Process') ;
#11521=PRODUCT_CONTEXT('part definition',#11520,'mechanical') ;
#11523=PRODUCT('Latch Housing with Base Plate (cast steel)',
'Latch Housing with Base Plate (cast steel)',$,(#11521)) ;
#11539=PRESENTATION_STYLE_ASSIGNMENT((#11555)) ;
#11555=SURFACE_STYLE_USAGE(.BOTH.,#11571) ;
#11571=SURFACE_SIDE_STYLE('',(#11587)) ;
#11587=SURFACE_STYLE_FILL_AREA(#11603) ;
#11603=FILL_AREA_STYLE(
'MAS-252 Grey Paint - Latch Housing with Base Plate (cast stee',(#11619)) ;
#11619=FILL_AREA_STYLE_COLOUR(
'MAS-252 Grey Paint - Latch Housing with Base Plate (cast stee',#11635) ;
#11635=COLOUR_RGB(
'MAS-252 Grey Paint - Latch Housing with Base Plate (cast stee', 0.09019608, 0.27058824, 0.51372549) ;
ENDSEC;
END-ISO-10303-21;
